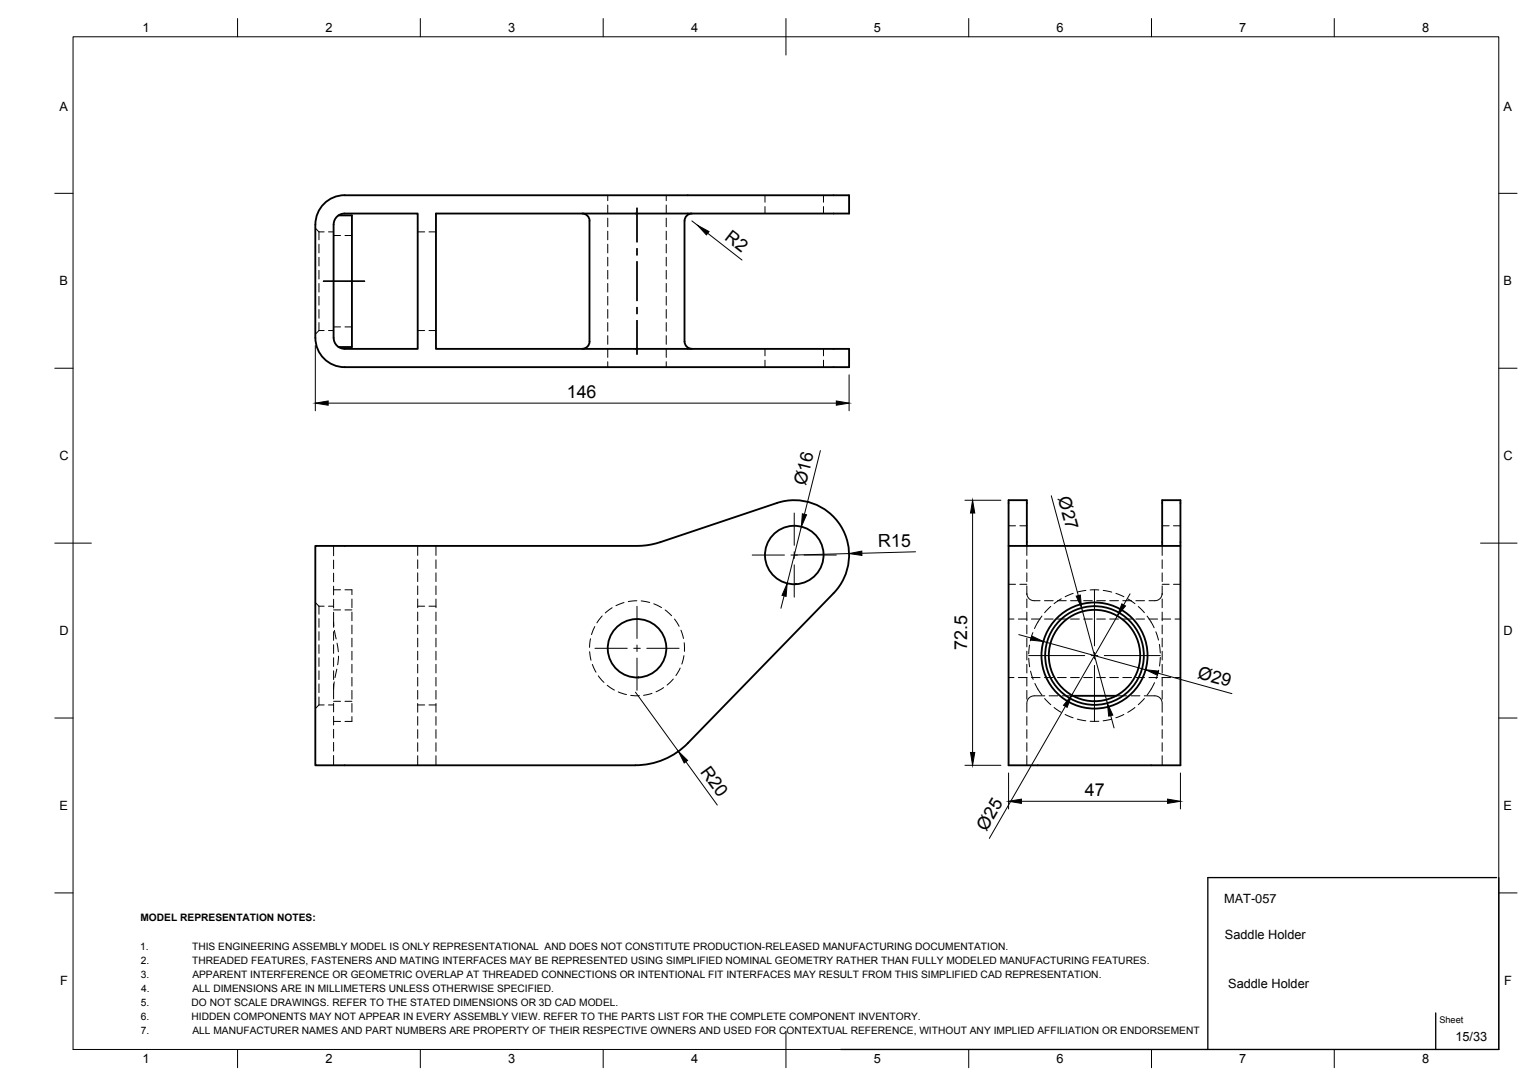
ISO-10303-21;
HEADER;
/* Generated by software containing ST-Developer
 * from STEP Tools, Inc. (www.steptools.com) 
 */

FILE_DESCRIPTION(
/* description */ ('STEP AP214', 'CAx-IF Rec.Pracs.---Representation and Presentation of Product Manufa
cturing Information (PMI)---4.0---2014-10-13'),
/* implementation_level */ '2;1');

FILE_NAME(
/* name */ 'Saddle Holder.step',
/* time_stamp */ '2026-10-28T23:34:22+01:00',
/* author */ (''),
/* organization */ (''),
/* preprocessor_version */ 'ST-DEVELOPER v20.2',
/* originating_system */ 'Autodesk Translation Framework v15.17.0.0',
/* authorisation */ '');

FILE_SCHEMA (('AP242_MANAGED_MODEL_BASED_3D_ENGINEERING_MIM_LF { 1 0 10303 442 2 1 4 }'));
ENDSEC;

DATA;
#10=MECHANICAL_DESIGN_GEOMETRIC_PRESENTATION_REPRESENTATION('',(#255),#27807);
#210=SHAPE_REPRESENTATION_RELATIONSHIP('SRR','None',#27906,#232);
#232=ADVANCED_BREP_SHAPE_REPRESENTATION('',(#284),#27786);
#255=STYLED_ITEM('',(#28091),#284);
#284=MANIFOLD_SOLID_BREP('Body1',#12031);
#378=FACE_BOUND('',#2260,.T.);
#379=FACE_BOUND('',#2261,.T.);
#380=FACE_BOUND('',#2263,.T.);
#381=FACE_BOUND('',#2264,.T.);
#382=FACE_BOUND('',#2266,.T.);
#383=FACE_BOUND('',#2268,.T.);
#384=FACE_BOUND('',#2272,.T.);
#385=FACE_BOUND('',#2276,.T.);
#386=FACE_BOUND('',#2278,.T.);
#387=FACE_BOUND('',#2279,.T.);
#388=FACE_BOUND('',#2281,.T.);
#389=FACE_BOUND('',#2282,.T.);
#390=FACE_BOUND('',#2284,.T.);
#391=FACE_BOUND('',#2289,.T.);
#392=FACE_BOUND('',#2291,.T.);
#559=PLANE('',#12904);
#560=PLANE('',#12908);
#561=PLANE('',#12909);
#562=PLANE('',#12910);
#563=PLANE('',#12913);
#564=PLANE('',#12916);
#565=PLANE('',#12917);
#566=PLANE('',#12920);
#567=PLANE('',#12921);
#568=PLANE('',#12922);
#569=PLANE('',#12927);
#570=PLANE('',#12928);
#571=PLANE('',#12931);
#572=PLANE('',#12934);
#573=PLANE('',#12935);
#574=PLANE('',#12936);
#575=PLANE('',#12937);
#576=PLANE('',#12938);
#577=PLANE('',#12939);
#827=TOROIDAL_SURFACE('',#12863,15.,2.);
#828=TOROIDAL_SURFACE('',#12868,15.,2.);
#874=B_SPLINE_CURVE_WITH_KNOTS('',3,(#19078,#19079,#19080,#19081,#19082,
#19083,#19084,#19085,#19086,#19087,#19088,#19089,#19090,#19091),
 .UNSPECIFIED.,.F.,.F.,(4,2,2,2,2,2,4),(2.17202184366925,2.28922044415962,
2.56626725236737,3.12036086878288,3.67445448519838,3.95150129340613,4.06869989389652),
 .UNSPECIFIED.);
#875=B_SPLINE_CURVE_WITH_KNOTS('',3,(#19095,#19096,#19097,#19098,#19099,
#19100,#19101,#19102),.UNSPECIFIED.,.F.,.F.,(4,2,2,4),(-0.94833902511363,
-0.831140424623256,-0.554093616415504,0.),.UNSPECIFIED.);
#876=B_SPLINE_CURVE_WITH_KNOTS('',3,(#19107,#19108,#19109,#19110,#19111,
#19112,#19113,#19114),.UNSPECIFIED.,.F.,.F.,(4,2,2,4),(0.,0.554093616415503,
0.831140424623253,0.948339025113634),.UNSPECIFIED.);
#1073=CYLINDRICAL_SURFACE('',#12873,13.);
#1074=CYLINDRICAL_SURFACE('',#12874,12.5);
#1075=CYLINDRICAL_SURFACE('',#12877,18.);
#1076=CYLINDRICAL_SURFACE('',#12881,13.5);
#1077=CYLINDRICAL_SURFACE('',#12884,13.5);
#1078=CYLINDRICAL_SURFACE('',#12886,8.00000000000002);
#1079=CYLINDRICAL_SURFACE('',#12889,8.00000000000002);
#1080=CYLINDRICAL_SURFACE('',#12892,15.);
#1081=CYLINDRICAL_SURFACE('',#12895,8.00000000000002);
#1082=CYLINDRICAL_SURFACE('',#12898,15.);
#1083=CYLINDRICAL_SURFACE('',#12901,3.);
#1084=CYLINDRICAL_SURFACE('',#12905,3.);
#1085=CYLINDRICAL_SURFACE('',#12925,8.00000000000001);
#1086=CYLINDRICAL_SURFACE('',#12926,8.00000000000001);
#1087=CYLINDRICAL_SURFACE('',#12940,20.);
#1088=CYLINDRICAL_SURFACE('',#12941,20.);
#1089=CYLINDRICAL_SURFACE('',#12942,20.);
#1090=CYLINDRICAL_SURFACE('',#12943,20.);
#1501=FACE_OUTER_BOUND('',#2241,.T.);
#1502=FACE_OUTER_BOUND('',#2242,.T.);
#1503=FACE_OUTER_BOUND('',#2243,.T.);
#1504=FACE_OUTER_BOUND('',#2244,.T.);
#1505=FACE_OUTER_BOUND('',#2245,.T.);
#1506=FACE_OUTER_BOUND('',#2246,.T.);
#1507=FACE_OUTER_BOUND('',#2247,.T.);
#1508=FACE_OUTER_BOUND('',#2248,.T.);
#1509=FACE_OUTER_BOUND('',#2249,.T.);
#1510=FACE_OUTER_BOUND('',#2250,.T.);
#1511=FACE_OUTER_BOUND('',#2251,.T.);
#1512=FACE_OUTER_BOUND('',#2252,.T.);
#1513=FACE_OUTER_BOUND('',#2253,.T.);
#1514=FACE_OUTER_BOUND('',#2254,.T.);
#1515=FACE_OUTER_BOUND('',#2255,.T.);
#1516=FACE_OUTER_BOUND('',#2256,.T.);
#1517=FACE_OUTER_BOUND('',#2257,.T.);
#1518=FACE_OUTER_BOUND('',#2258,.T.);
#1519=FACE_OUTER_BOUND('',#2259,.T.);
#1520=FACE_OUTER_BOUND('',#2262,.T.);
#1521=FACE_OUTER_BOUND('',#2265,.T.);
#1522=FACE_OUTER_BOUND('',#2267,.T.);
#1523=FACE_OUTER_BOUND('',#2269,.T.);
#1524=FACE_OUTER_BOUND('',#2270,.T.);
#1525=FACE_OUTER_BOUND('',#2271,.T.);
#1526=FACE_OUTER_BOUND('',#2273,.T.);
#1527=FACE_OUTER_BOUND('',#2274,.T.);
#1528=FACE_OUTER_BOUND('',#2275,.T.);
#1529=FACE_OUTER_BOUND('',#2277,.T.);
#1530=FACE_OUTER_BOUND('',#2280,.T.);
#1531=FACE_OUTER_BOUND('',#2283,.T.);
#1532=FACE_OUTER_BOUND('',#2285,.T.);
#1533=FACE_OUTER_BOUND('',#2286,.T.);
#1534=FACE_OUTER_BOUND('',#2287,.T.);
#1535=FACE_OUTER_BOUND('',#2288,.T.);
#1536=FACE_OUTER_BOUND('',#2290,.T.);
#1537=FACE_OUTER_BOUND('',#2292,.T.);
#1538=FACE_OUTER_BOUND('',#2293,.T.);
#1539=FACE_OUTER_BOUND('',#2294,.T.);
#1540=FACE_OUTER_BOUND('',#2295,.T.);
#2241=EDGE_LOOP('',(#9169,#9170,#9171,#9172));
#2242=EDGE_LOOP('',(#9173,#9174,#9175,#9176,#9177));
#2243=EDGE_LOOP('',(#9178,#9179,#9180,#9181,#9182));
#2244=EDGE_LOOP('',(#9183,#9184,#9185,#9186,#9187,#9188));
#2245=EDGE_LOOP('',(#9189,#9190,#9191,#9192));
#2246=EDGE_LOOP('',(#9193,#9194,#9195,#9196,#9197,#9198,#9199,#9200));
#2247=EDGE_LOOP('',(#9201,#9202,#9203,#9204));
#2248=EDGE_LOOP('',(#9205,#9206,#9207,#9208));
#2249=EDGE_LOOP('',(#9209,#9210,#9211,#9212));
#2250=EDGE_LOOP('',(#9213,#9214,#9215,#9216));
#2251=EDGE_LOOP('',(#9217,#9218,#9219,#9220));
#2252=EDGE_LOOP('',(#9221,#9222,#9223,#9224));
#2253=EDGE_LOOP('',(#9225,#9226,#9227,#9228));
#2254=EDGE_LOOP('',(#9229,#9230,#9231,#9232,#9233,#9234));
#2255=EDGE_LOOP('',(#9235,#9236,#9237,#9238));
#2256=EDGE_LOOP('',(#9239,#9240,#9241,#9242,#9243,#9244,#9245));
#2257=EDGE_LOOP('',(#9246,#9247,#9248,#9249));
#2258=EDGE_LOOP('',(#9250,#9251,#9252,#9253));
#2259=EDGE_LOOP('',(#9254,#9255,#9256,#9257,#9258,#9259,#9260,#9261));
#2260=EDGE_LOOP('',(#9262));
#2261=EDGE_LOOP('',(#9263));
#2262=EDGE_LOOP('',(#9264,#9265,#9266,#9267,#9268,#9269,#9270,#9271));
#2263=EDGE_LOOP('',(#9272));
#2264=EDGE_LOOP('',(#9273));
#2265=EDGE_LOOP('',(#9274,#9275,#9276,#9277));
#2266=EDGE_LOOP('',(#9278));
#2267=EDGE_LOOP('',(#9279,#9280,#9281,#9282,#9283,#9284,#9285,#9286,#9287,
#9288));
#2268=EDGE_LOOP('',(#9289,#9290,#9291,#9292,#9293,#9294));
#2269=EDGE_LOOP('',(#9295,#9296,#9297,#9298));
#2270=EDGE_LOOP('',(#9299,#9300,#9301,#9302));
#2271=EDGE_LOOP('',(#9303,#9304,#9305,#9306,#9307,#9308,#9309,#9310,#9311,
#9312));
#2272=EDGE_LOOP('',(#9313,#9314,#9315,#9316,#9317,#9318));
#2273=EDGE_LOOP('',(#9319,#9320,#9321,#9322));
#2274=EDGE_LOOP('',(#9323,#9324,#9325,#9326));
#2275=EDGE_LOOP('',(#9327,#9328,#9329,#9330));
#2276=EDGE_LOOP('',(#9331));
#2277=EDGE_LOOP('',(#9332,#9333,#9334,#9335,#9336,#9337,#9338,#9339));
#2278=EDGE_LOOP('',(#9340));
#2279=EDGE_LOOP('',(#9341));
#2280=EDGE_LOOP('',(#9342,#9343,#9344,#9345,#9346,#9347,#9348,#9349));
#2281=EDGE_LOOP('',(#9350));
#2282=EDGE_LOOP('',(#9351));
#2283=EDGE_LOOP('',(#9352,#9353,#9354,#9355));
#2284=EDGE_LOOP('',(#9356));
#2285=EDGE_LOOP('',(#9357,#9358,#9359,#9360));
#2286=EDGE_LOOP('',(#9361,#9362,#9363,#9364));
#2287=EDGE_LOOP('',(#9365,#9366,#9367,#9368));
#2288=EDGE_LOOP('',(#9369));
#2289=EDGE_LOOP('',(#9370));
#2290=EDGE_LOOP('',(#9371));
#2291=EDGE_LOOP('',(#9372));
#2292=EDGE_LOOP('',(#9373,#9374,#9375,#9376));
#2293=EDGE_LOOP('',(#9377,#9378,#9379,#9380));
#2294=EDGE_LOOP('',(#9381,#9382,#9383,#9384));
#2295=EDGE_LOOP('',(#9385,#9386,#9387,#9388));
#3073=LINE('',#19049,#3893);
#3074=LINE('',#19068,#3894);
#3075=LINE('',#19073,#3895);
#3076=LINE('',#19104,#3896);
#3077=LINE('',#19120,#3897);
#3078=LINE('',#19125,#3898);
#3079=LINE('',#19130,#3899);
#3080=LINE('',#19136,#3900);
#3081=LINE('',#19143,#3901);
#3082=LINE('',#19146,#3902);
#3083=LINE('',#19151,#3903);
#3084=LINE('',#19158,#3904);
#3085=LINE('',#19161,#3905);
#3086=LINE('',#19164,#3906);
#3087=LINE('',#19168,#3907);
#3088=LINE('',#19171,#3908);
#3089=LINE('',#19174,#3909);
#3090=LINE('',#19175,#3910);
#3091=LINE('',#19180,#3911);
#3092=LINE('',#19183,#3912);
#3093=LINE('',#19186,#3913);
#3094=LINE('',#19188,#3914);
#3095=LINE('',#19189,#3915);
#3096=LINE('',#19192,#3916);
#3097=LINE('',#19194,#3917);
#3098=LINE('',#19195,#3918);
#3099=LINE('',#19198,#3919);
#3100=LINE('',#19202,#3920);
#3101=LINE('',#19204,#3921);
#3102=LINE('',#19206,#3922);
#3103=LINE('',#19209,#3923);
#3104=LINE('',#19213,#3924);
#3105=LINE('',#19218,#3925);
#3106=LINE('',#19219,#3926);
#3107=LINE('',#19223,#3927);
#3108=LINE('',#19225,#3928);
#3109=LINE('',#19227,#3929);
#3110=LINE('',#19228,#3930);
#3111=LINE('',#19232,#3931);
#3112=LINE('',#19233,#3932);
#3113=LINE('',#19237,#3933);
#3114=LINE('',#19239,#3934);
#3115=LINE('',#19240,#3935);
#3116=LINE('',#19242,#3936);
#3117=LINE('',#19244,#3937);
#3118=LINE('',#19245,#3938);
#3119=LINE('',#19248,#3939);
#3120=LINE('',#19249,#3940);
#3121=LINE('',#19252,#3941);
#3122=LINE('',#19253,#3942);
#3123=LINE('',#19257,#3943);
#3124=LINE('',#19258,#3944);
#3125=LINE('',#19262,#3945);
#3126=LINE('',#19264,#3946);
#3127=LINE('',#19265,#3947);
#3128=LINE('',#19267,#3948);
#3129=LINE('',#19269,#3949);
#3130=LINE('',#19270,#3950);
#3131=LINE('',#19271,#3951);
#3132=LINE('',#19275,#3952);
#3133=LINE('',#19276,#3953);
#3134=LINE('',#19284,#3954);
#3135=LINE('',#19285,#3955);
#3893=VECTOR('',#15179,13.5);
#3894=VECTOR('',#15204,13.);
#3895=VECTOR('',#15209,12.5);
#3896=VECTOR('',#15216,18.);
#3897=VECTOR('',#15225,13.5);
#3898=VECTOR('',#15232,13.5);
#3899=VECTOR('',#15237,8.00000000000002);
#3900=VECTOR('',#15244,8.00000000000002);
#3901=VECTOR('',#15251,1000.);
#3902=VECTOR('',#15254,1000.);
#3903=VECTOR('',#15259,8.00000000000002);
#3904=VECTOR('',#15266,1000.);
#3905=VECTOR('',#15269,1000.);
#3906=VECTOR('',#15272,1000.);
#3907=VECTOR('',#15275,1000.);
#3908=VECTOR('',#15278,1000.);
#3909=VECTOR('',#15281,1000.);
#3910=VECTOR('',#15282,1000.);
#3911=VECTOR('',#15287,1000.);
#3912=VECTOR('',#15290,1000.);
#3913=VECTOR('',#15293,1000.);
#3914=VECTOR('',#15294,1000.);
#3915=VECTOR('',#15295,1000.);
#3916=VECTOR('',#15298,1000.);
#3917=VECTOR('',#15299,1000.);
#3918=VECTOR('',#15300,1000.);
#3919=VECTOR('',#15303,1000.);
#3920=VECTOR('',#15306,1000.);
#3921=VECTOR('',#15307,1000.);
#3922=VECTOR('',#15308,1000.);
#3923=VECTOR('',#15311,1000.);
#3924=VECTOR('',#15314,1000.);
#3925=VECTOR('',#15319,1000.);
#3926=VECTOR('',#15320,1000.);
#3927=VECTOR('',#15323,1000.);
#3928=VECTOR('',#15324,1000.);
#3929=VECTOR('',#15325,1000.);
#3930=VECTOR('',#15326,1000.);
#3931=VECTOR('',#15329,1000.);
#3932=VECTOR('',#15330,1000.);
#3933=VECTOR('',#15335,1000.);
#3934=VECTOR('',#15336,1000.);
#3935=VECTOR('',#15337,1000.);
#3936=VECTOR('',#15338,1000.);
#3937=VECTOR('',#15339,1000.);
#3938=VECTOR('',#15340,1000.);
#3939=VECTOR('',#15343,1000.);
#3940=VECTOR('',#15344,1000.);
#3941=VECTOR('',#15347,1000.);
#3942=VECTOR('',#15348,1000.);
#3943=VECTOR('',#15351,1000.);
#3944=VECTOR('',#15352,1000.);
#3945=VECTOR('',#15357,1000.);
#3946=VECTOR('',#15358,1000.);
#3947=VECTOR('',#15359,1000.);
#3948=VECTOR('',#15360,1000.);
#3949=VECTOR('',#15361,1000.);
#3950=VECTOR('',#15362,1000.);
#3951=VECTOR('',#15363,1000.);
#3952=VECTOR('',#15370,1000.);
#3953=VECTOR('',#15371,1000.);
#3954=VECTOR('',#15386,1000.);
#3955=VECTOR('',#15387,1000.);
#4669=CIRCLE('',#12861,13.5);
#4670=CIRCLE('',#12862,14.5);
#4671=CIRCLE('',#12864,15.);
#4672=CIRCLE('',#12865,2.);
#4673=CIRCLE('',#12866,13.);
#4674=CIRCLE('',#12867,13.);
#4675=CIRCLE('',#12869,15.);
#4676=CIRCLE('',#12870,2.);
#4677=CIRCLE('',#12871,13.);
#4678=CIRCLE('',#12872,13.);
#4679=CIRCLE('',#12875,12.5);
#4680=CIRCLE('',#12876,12.5);
#4681=CIRCLE('',#12878,18.);
#4682=CIRCLE('',#12879,18.);
#4683=CIRCLE('',#12880,18.);
#4684=CIRCLE('',#12882,13.5);
#4685=CIRCLE('',#12883,13.5);
#4686=CIRCLE('',#12885,13.5);
#4687=CIRCLE('',#12887,8.00000000000002);
#4688=CIRCLE('',#12888,8.00000000000002);
#4689=CIRCLE('',#12890,8.00000000000002);
#4690=CIRCLE('',#12891,8.);
#4691=CIRCLE('',#12893,15.);
#4692=CIRCLE('',#12894,15.);
#4693=CIRCLE('',#12896,7.99999999999999);
#4694=CIRCLE('',#12897,8.00000000000002);
#4695=CIRCLE('',#12899,15.);
#4696=CIRCLE('',#12900,15.);
#4697=CIRCLE('',#12902,3.);
#4698=CIRCLE('',#12903,2.99999999999999);
#4699=CIRCLE('',#12906,2.99999999999999);
#4700=CIRCLE('',#12907,3.);
#4701=CIRCLE('',#12911,20.);
#4702=CIRCLE('',#12912,20.);
#4703=CIRCLE('',#12914,20.);
#4704=CIRCLE('',#12915,20.);
#4705=CIRCLE('',#12918,8.00000000000002);
#4706=CIRCLE('',#12919,8.00000000000002);
#4707=CIRCLE('',#12923,8.00000000000001);
#4708=CIRCLE('',#12924,8.00000000000001);
#4709=CIRCLE('',#12929,20.);
#4710=CIRCLE('',#12930,20.);
#4711=CIRCLE('',#12932,20.);
#4712=CIRCLE('',#12933,20.);
#5461=VERTEX_POINT('',#19046);
#5462=VERTEX_POINT('',#19048);
#5463=VERTEX_POINT('',#19052);
#5464=VERTEX_POINT('',#19054);
#5465=VERTEX_POINT('',#19056);
#5466=VERTEX_POINT('',#19060);
#5467=VERTEX_POINT('',#19062);
#5468=VERTEX_POINT('',#19064);
#5469=VERTEX_POINT('',#19070);
#5470=VERTEX_POINT('',#19072);
#5471=VERTEX_POINT('',#19076);
#5472=VERTEX_POINT('',#19077);
#5473=VERTEX_POINT('',#19092);
#5474=VERTEX_POINT('',#19094);
#5475=VERTEX_POINT('',#19103);
#5476=VERTEX_POINT('',#19106);
#5477=VERTEX_POINT('',#19117);
#5478=VERTEX_POINT('',#19119);
#5479=VERTEX_POINT('',#19123);
#5480=VERTEX_POINT('',#19127);
#5481=VERTEX_POINT('',#19129);
#5482=VERTEX_POINT('',#19133);
#5483=VERTEX_POINT('',#19135);
#5484=VERTEX_POINT('',#19139);
#5485=VERTEX_POINT('',#19140);
#5486=VERTEX_POINT('',#19142);
#5487=VERTEX_POINT('',#19144);
#5488=VERTEX_POINT('',#19148);
#5489=VERTEX_POINT('',#19150);
#5490=VERTEX_POINT('',#19154);
#5491=VERTEX_POINT('',#19155);
#5492=VERTEX_POINT('',#19157);
#5493=VERTEX_POINT('',#19159);
#5494=VERTEX_POINT('',#19163);
#5495=VERTEX_POINT('',#19165);
#5496=VERTEX_POINT('',#19167);
#5497=VERTEX_POINT('',#19169);
#5498=VERTEX_POINT('',#19173);
#5499=VERTEX_POINT('',#19177);
#5500=VERTEX_POINT('',#19179);
#5501=VERTEX_POINT('',#19181);
#5502=VERTEX_POINT('',#19185);
#5503=VERTEX_POINT('',#19187);
#5504=VERTEX_POINT('',#19191);
#5505=VERTEX_POINT('',#19193);
#5506=VERTEX_POINT('',#19197);
#5507=VERTEX_POINT('',#19199);
#5508=VERTEX_POINT('',#19201);
#5509=VERTEX_POINT('',#19203);
#5510=VERTEX_POINT('',#19205);
#5511=VERTEX_POINT('',#19207);
#5512=VERTEX_POINT('',#19211);
#5513=VERTEX_POINT('',#19212);
#5514=VERTEX_POINT('',#19215);
#5515=VERTEX_POINT('',#19217);
#5516=VERTEX_POINT('',#19221);
#5517=VERTEX_POINT('',#19222);
#5518=VERTEX_POINT('',#19224);
#5519=VERTEX_POINT('',#19226);
#5520=VERTEX_POINT('',#19230);
#5521=VERTEX_POINT('',#19231);
#5522=VERTEX_POINT('',#19236);
#5523=VERTEX_POINT('',#19238);
#5524=VERTEX_POINT('',#19241);
#5525=VERTEX_POINT('',#19243);
#5526=VERTEX_POINT('',#19247);
#5527=VERTEX_POINT('',#19251);
#5528=VERTEX_POINT('',#19255);
#5529=VERTEX_POINT('',#19256);
#5530=VERTEX_POINT('',#19261);
#5531=VERTEX_POINT('',#19263);
#5532=VERTEX_POINT('',#19266);
#5533=VERTEX_POINT('',#19268);
#6797=EDGE_CURVE('',#5461,#5461,#4669,.T.);
#6798=EDGE_CURVE('',#5461,#5462,#3073,.T.);
#6799=EDGE_CURVE('',#5462,#5462,#4670,.T.);
#6800=EDGE_CURVE('',#5463,#5463,#4671,.T.);
#6801=EDGE_CURVE('',#5463,#5464,#4672,.T.);
#6802=EDGE_CURVE('',#5465,#5464,#4673,.T.);
#6803=EDGE_CURVE('',#5464,#5465,#4674,.T.);
#6804=EDGE_CURVE('',#5466,#5466,#4675,.T.);
#6805=EDGE_CURVE('',#5466,#5467,#4676,.T.);
#6806=EDGE_CURVE('',#5468,#5467,#4677,.T.);
#6807=EDGE_CURVE('',#5467,#5468,#4678,.T.);
#6808=EDGE_CURVE('',#5465,#5468,#3074,.T.);
#6809=EDGE_CURVE('',#5469,#5469,#4679,.T.);
#6810=EDGE_CURVE('',#5469,#5470,#3075,.T.);
#6811=EDGE_CURVE('',#5470,#5470,#4680,.T.);
#6812=EDGE_CURVE('',#5471,#5472,#874,.F.);
#6813=EDGE_CURVE('',#5472,#5473,#4681,.T.);
#6814=EDGE_CURVE('',#5473,#5474,#875,.T.);
#6815=EDGE_CURVE('',#5474,#5475,#3076,.T.);
#6816=EDGE_CURVE('',#5475,#5475,#4682,.T.);
#6817=EDGE_CURVE('',#5474,#5476,#876,.T.);
#6818=EDGE_CURVE('',#5476,#5471,#4683,.T.);
#6819=EDGE_CURVE('',#5477,#5477,#4684,.T.);
#6820=EDGE_CURVE('',#5477,#5478,#3077,.T.);
#6821=EDGE_CURVE('',#5478,#5478,#4685,.T.);
#6822=EDGE_CURVE('',#5479,#5479,#4686,.T.);
#6823=EDGE_CURVE('',#5479,#5461,#3078,.T.);
#6824=EDGE_CURVE('',#5480,#5480,#4687,.T.);
#6825=EDGE_CURVE('',#5480,#5481,#3079,.T.);
#6826=EDGE_CURVE('',#5481,#5481,#4688,.T.);
#6827=EDGE_CURVE('',#5482,#5482,#4689,.T.);
#6828=EDGE_CURVE('',#5482,#5483,#3080,.T.);
#6829=EDGE_CURVE('',#5483,#5483,#4690,.T.);
#6830=EDGE_CURVE('',#5484,#5485,#4691,.T.);
#6831=EDGE_CURVE('',#5485,#5486,#3081,.T.);
#6832=EDGE_CURVE('',#5486,#5487,#4692,.T.);
#6833=EDGE_CURVE('',#5484,#5487,#3082,.T.);
#6834=EDGE_CURVE('',#5488,#5488,#4693,.T.);
#6835=EDGE_CURVE('',#5488,#5489,#3083,.T.);
#6836=EDGE_CURVE('',#5489,#5489,#4694,.T.);
#6837=EDGE_CURVE('',#5490,#5491,#4695,.T.);
#6838=EDGE_CURVE('',#5490,#5492,#3084,.T.);
#6839=EDGE_CURVE('',#5492,#5493,#4696,.T.);
#6840=EDGE_CURVE('',#5491,#5493,#3085,.T.);
#6841=EDGE_CURVE('',#5471,#5494,#3086,.T.);
#6842=EDGE_CURVE('',#5494,#5495,#4697,.T.);
#6843=EDGE_CURVE('',#5496,#5495,#3087,.T.);
#6844=EDGE_CURVE('',#5497,#5496,#4698,.T.);
#6845=EDGE_CURVE('',#5497,#5472,#3088,.T.);
#6846=EDGE_CURVE('',#5498,#5497,#3089,.T.);
#6847=EDGE_CURVE('',#5498,#5473,#3090,.T.);
#6848=EDGE_CURVE('',#5499,#5498,#4699,.T.);
#6849=EDGE_CURVE('',#5499,#5500,#3091,.T.);
#6850=EDGE_CURVE('',#5500,#5501,#4700,.T.);
#6851=EDGE_CURVE('',#5476,#5501,#3092,.T.);
#6852=EDGE_CURVE('',#5485,#5502,#3093,.T.);
#6853=EDGE_CURVE('',#5502,#5503,#3094,.T.);
#6854=EDGE_CURVE('',#5503,#5486,#3095,.T.);
#6855=EDGE_CURVE('',#5487,#5504,#3096,.T.);
#6856=EDGE_CURVE('',#5504,#5505,#3097,.T.);
#6857=EDGE_CURVE('',#5505,#5484,#3098,.T.);
#6858=EDGE_CURVE('',#5491,#5506,#3099,.T.);
#6859=EDGE_CURVE('',#5506,#5507,#4701,.T.);
#6860=EDGE_CURVE('',#5507,#5508,#3100,.T.);
#6861=EDGE_CURVE('',#5508,#5509,#3101,.T.);
#6862=EDGE_CURVE('',#5509,#5510,#3102,.T.);
#6863=EDGE_CURVE('',#5510,#5511,#4702,.T.);
#6864=EDGE_CURVE('',#5511,#5490,#3103,.T.);
#6865=EDGE_CURVE('',#5512,#5513,#3104,.T.);
#6866=EDGE_CURVE('',#5512,#5504,#4703,.T.);
#6867=EDGE_CURVE('',#5503,#5514,#4704,.T.);
#6868=EDGE_CURVE('',#5515,#5514,#3105,.T.);
#6869=EDGE_CURVE('',#5515,#5513,#3106,.T.);
#6870=EDGE_CURVE('',#5516,#5517,#3107,.T.);
#6871=EDGE_CURVE('',#5517,#5518,#3108,.T.);
#6872=EDGE_CURVE('',#5519,#5518,#3109,.T.);
#6873=EDGE_CURVE('',#5519,#5516,#3110,.T.);
#6874=EDGE_CURVE('',#5520,#5521,#3111,.T.);
#6875=EDGE_CURVE('',#5521,#5510,#3112,.T.);
#6876=EDGE_CURVE('',#5509,#5519,#4705,.T.);
#6877=EDGE_CURVE('',#5518,#5515,#4706,.T.);
#6878=EDGE_CURVE('',#5514,#5522,#3113,.T.);
#6879=EDGE_CURVE('',#5522,#5523,#3114,.T.);
#6880=EDGE_CURVE('',#5523,#5520,#3115,.T.);
#6881=EDGE_CURVE('',#5496,#5524,#3116,.T.);
#6882=EDGE_CURVE('',#5524,#5525,#3117,.T.);
#6883=EDGE_CURVE('',#5525,#5499,#3118,.T.);
#6884=EDGE_CURVE('',#5511,#5526,#3119,.T.);
#6885=EDGE_CURVE('',#5526,#5492,#3120,.T.);
#6886=EDGE_CURVE('',#5493,#5527,#3121,.T.);
#6887=EDGE_CURVE('',#5527,#5506,#3122,.T.);
#6888=EDGE_CURVE('',#5528,#5529,#3123,.T.);
#6889=EDGE_CURVE('',#5528,#5512,#3124,.T.);
#6890=EDGE_CURVE('',#5513,#5517,#4707,.T.);
#6891=EDGE_CURVE('',#5516,#5508,#4708,.T.);
#6892=EDGE_CURVE('',#5507,#5530,#3125,.T.);
#6893=EDGE_CURVE('',#5531,#5530,#3126,.T.);
#6894=EDGE_CURVE('',#5529,#5531,#3127,.T.);
#6895=EDGE_CURVE('',#5532,#5500,#3128,.T.);
#6896=EDGE_CURVE('',#5533,#5532,#3129,.T.);
#6897=EDGE_CURVE('',#5495,#5533,#3130,.T.);
#6898=EDGE_CURVE('',#5501,#5494,#3131,.T.);
#6899=EDGE_CURVE('',#5523,#5529,#3132,.T.);
#6900=EDGE_CURVE('',#5520,#5531,#3133,.T.);
#6901=EDGE_CURVE('',#5505,#5528,#4709,.T.);
#6902=EDGE_CURVE('',#5522,#5502,#4710,.T.);
#6903=EDGE_CURVE('',#5530,#5527,#4711,.T.);
#6904=EDGE_CURVE('',#5526,#5521,#4712,.T.);
#6905=EDGE_CURVE('',#5524,#5533,#3134,.T.);
#6906=EDGE_CURVE('',#5525,#5532,#3135,.T.);
#9169=ORIENTED_EDGE('',*,*,#6797,.F.);
#9170=ORIENTED_EDGE('',*,*,#6798,.T.);
#9171=ORIENTED_EDGE('',*,*,#6799,.F.);
#9172=ORIENTED_EDGE('',*,*,#6798,.F.);
#9173=ORIENTED_EDGE('',*,*,#6800,.F.);
#9174=ORIENTED_EDGE('',*,*,#6801,.T.);
#9175=ORIENTED_EDGE('',*,*,#6802,.F.);
#9176=ORIENTED_EDGE('',*,*,#6803,.F.);
#9177=ORIENTED_EDGE('',*,*,#6801,.F.);
#9178=ORIENTED_EDGE('',*,*,#6804,.F.);
#9179=ORIENTED_EDGE('',*,*,#6805,.T.);
#9180=ORIENTED_EDGE('',*,*,#6806,.F.);
#9181=ORIENTED_EDGE('',*,*,#6807,.F.);
#9182=ORIENTED_EDGE('',*,*,#6805,.F.);
#9183=ORIENTED_EDGE('',*,*,#6802,.T.);
#9184=ORIENTED_EDGE('',*,*,#6803,.T.);
#9185=ORIENTED_EDGE('',*,*,#6808,.T.);
#9186=ORIENTED_EDGE('',*,*,#6806,.T.);
#9187=ORIENTED_EDGE('',*,*,#6807,.T.);
#9188=ORIENTED_EDGE('',*,*,#6808,.F.);
#9189=ORIENTED_EDGE('',*,*,#6809,.T.);
#9190=ORIENTED_EDGE('',*,*,#6810,.T.);
#9191=ORIENTED_EDGE('',*,*,#6811,.F.);
#9192=ORIENTED_EDGE('',*,*,#6810,.F.);
#9193=ORIENTED_EDGE('',*,*,#6812,.T.);
#9194=ORIENTED_EDGE('',*,*,#6813,.T.);
#9195=ORIENTED_EDGE('',*,*,#6814,.T.);
#9196=ORIENTED_EDGE('',*,*,#6815,.T.);
#9197=ORIENTED_EDGE('',*,*,#6816,.F.);
#9198=ORIENTED_EDGE('',*,*,#6815,.F.);
#9199=ORIENTED_EDGE('',*,*,#6817,.T.);
#9200=ORIENTED_EDGE('',*,*,#6818,.T.);
#9201=ORIENTED_EDGE('',*,*,#6819,.T.);
#9202=ORIENTED_EDGE('',*,*,#6820,.T.);
#9203=ORIENTED_EDGE('',*,*,#6821,.F.);
#9204=ORIENTED_EDGE('',*,*,#6820,.F.);
#9205=ORIENTED_EDGE('',*,*,#6822,.F.);
#9206=ORIENTED_EDGE('',*,*,#6823,.T.);
#9207=ORIENTED_EDGE('',*,*,#6797,.T.);
#9208=ORIENTED_EDGE('',*,*,#6823,.F.);
#9209=ORIENTED_EDGE('',*,*,#6824,.T.);
#9210=ORIENTED_EDGE('',*,*,#6825,.T.);
#9211=ORIENTED_EDGE('',*,*,#6826,.F.);
#9212=ORIENTED_EDGE('',*,*,#6825,.F.);
#9213=ORIENTED_EDGE('',*,*,#6827,.T.);
#9214=ORIENTED_EDGE('',*,*,#6828,.T.);
#9215=ORIENTED_EDGE('',*,*,#6829,.F.);
#9216=ORIENTED_EDGE('',*,*,#6828,.F.);
#9217=ORIENTED_EDGE('',*,*,#6830,.T.);
#9218=ORIENTED_EDGE('',*,*,#6831,.T.);
#9219=ORIENTED_EDGE('',*,*,#6832,.T.);
#9220=ORIENTED_EDGE('',*,*,#6833,.F.);
#9221=ORIENTED_EDGE('',*,*,#6834,.F.);
#9222=ORIENTED_EDGE('',*,*,#6835,.T.);
#9223=ORIENTED_EDGE('',*,*,#6836,.F.);
#9224=ORIENTED_EDGE('',*,*,#6835,.F.);
#9225=ORIENTED_EDGE('',*,*,#6837,.F.);
#9226=ORIENTED_EDGE('',*,*,#6838,.T.);
#9227=ORIENTED_EDGE('',*,*,#6839,.T.);
#9228=ORIENTED_EDGE('',*,*,#6840,.F.);
#9229=ORIENTED_EDGE('',*,*,#6812,.F.);
#9230=ORIENTED_EDGE('',*,*,#6841,.T.);
#9231=ORIENTED_EDGE('',*,*,#6842,.T.);
#9232=ORIENTED_EDGE('',*,*,#6843,.F.);
#9233=ORIENTED_EDGE('',*,*,#6844,.F.);
#9234=ORIENTED_EDGE('',*,*,#6845,.T.);
#9235=ORIENTED_EDGE('',*,*,#6813,.F.);
#9236=ORIENTED_EDGE('',*,*,#6845,.F.);
#9237=ORIENTED_EDGE('',*,*,#6846,.F.);
#9238=ORIENTED_EDGE('',*,*,#6847,.T.);
#9239=ORIENTED_EDGE('',*,*,#6814,.F.);
#9240=ORIENTED_EDGE('',*,*,#6847,.F.);
#9241=ORIENTED_EDGE('',*,*,#6848,.F.);
#9242=ORIENTED_EDGE('',*,*,#6849,.T.);
#9243=ORIENTED_EDGE('',*,*,#6850,.T.);
#9244=ORIENTED_EDGE('',*,*,#6851,.F.);
#9245=ORIENTED_EDGE('',*,*,#6817,.F.);
#9246=ORIENTED_EDGE('',*,*,#6852,.T.);
#9247=ORIENTED_EDGE('',*,*,#6853,.T.);
#9248=ORIENTED_EDGE('',*,*,#6854,.T.);
#9249=ORIENTED_EDGE('',*,*,#6831,.F.);
#9250=ORIENTED_EDGE('',*,*,#6855,.T.);
#9251=ORIENTED_EDGE('',*,*,#6856,.T.);
#9252=ORIENTED_EDGE('',*,*,#6857,.T.);
#9253=ORIENTED_EDGE('',*,*,#6833,.T.);
#9254=ORIENTED_EDGE('',*,*,#6858,.T.);
#9255=ORIENTED_EDGE('',*,*,#6859,.T.);
#9256=ORIENTED_EDGE('',*,*,#6860,.T.);
#9257=ORIENTED_EDGE('',*,*,#6861,.T.);
#9258=ORIENTED_EDGE('',*,*,#6862,.T.);
#9259=ORIENTED_EDGE('',*,*,#6863,.T.);
#9260=ORIENTED_EDGE('',*,*,#6864,.T.);
#9261=ORIENTED_EDGE('',*,*,#6837,.T.);
#9262=ORIENTED_EDGE('',*,*,#6824,.F.);
#9263=ORIENTED_EDGE('',*,*,#6827,.F.);
#9264=ORIENTED_EDGE('',*,*,#6865,.F.);
#9265=ORIENTED_EDGE('',*,*,#6866,.T.);
#9266=ORIENTED_EDGE('',*,*,#6855,.F.);
#9267=ORIENTED_EDGE('',*,*,#6832,.F.);
#9268=ORIENTED_EDGE('',*,*,#6854,.F.);
#9269=ORIENTED_EDGE('',*,*,#6867,.T.);
#9270=ORIENTED_EDGE('',*,*,#6868,.F.);
#9271=ORIENTED_EDGE('',*,*,#6869,.T.);
#9272=ORIENTED_EDGE('',*,*,#6836,.T.);
#9273=ORIENTED_EDGE('',*,*,#6826,.T.);
#9274=ORIENTED_EDGE('',*,*,#6870,.T.);
#9275=ORIENTED_EDGE('',*,*,#6871,.T.);
#9276=ORIENTED_EDGE('',*,*,#6872,.F.);
#9277=ORIENTED_EDGE('',*,*,#6873,.T.);
#9278=ORIENTED_EDGE('',*,*,#6799,.T.);
#9279=ORIENTED_EDGE('',*,*,#6874,.T.);
#9280=ORIENTED_EDGE('',*,*,#6875,.T.);
#9281=ORIENTED_EDGE('',*,*,#6862,.F.);
#9282=ORIENTED_EDGE('',*,*,#6876,.T.);
#9283=ORIENTED_EDGE('',*,*,#6872,.T.);
#9284=ORIENTED_EDGE('',*,*,#6877,.T.);
#9285=ORIENTED_EDGE('',*,*,#6868,.T.);
#9286=ORIENTED_EDGE('',*,*,#6878,.T.);
#9287=ORIENTED_EDGE('',*,*,#6879,.T.);
#9288=ORIENTED_EDGE('',*,*,#6880,.T.);
#9289=ORIENTED_EDGE('',*,*,#6881,.T.);
#9290=ORIENTED_EDGE('',*,*,#6882,.T.);
#9291=ORIENTED_EDGE('',*,*,#6883,.T.);
#9292=ORIENTED_EDGE('',*,*,#6848,.T.);
#9293=ORIENTED_EDGE('',*,*,#6846,.T.);
#9294=ORIENTED_EDGE('',*,*,#6844,.T.);
#9295=ORIENTED_EDGE('',*,*,#6864,.F.);
#9296=ORIENTED_EDGE('',*,*,#6884,.T.);
#9297=ORIENTED_EDGE('',*,*,#6885,.T.);
#9298=ORIENTED_EDGE('',*,*,#6838,.F.);
#9299=ORIENTED_EDGE('',*,*,#6886,.T.);
#9300=ORIENTED_EDGE('',*,*,#6887,.T.);
#9301=ORIENTED_EDGE('',*,*,#6858,.F.);
#9302=ORIENTED_EDGE('',*,*,#6840,.T.);
#9303=ORIENTED_EDGE('',*,*,#6888,.F.);
#9304=ORIENTED_EDGE('',*,*,#6889,.T.);
#9305=ORIENTED_EDGE('',*,*,#6865,.T.);
#9306=ORIENTED_EDGE('',*,*,#6890,.T.);
#9307=ORIENTED_EDGE('',*,*,#6870,.F.);
#9308=ORIENTED_EDGE('',*,*,#6891,.T.);
#9309=ORIENTED_EDGE('',*,*,#6860,.F.);
#9310=ORIENTED_EDGE('',*,*,#6892,.T.);
#9311=ORIENTED_EDGE('',*,*,#6893,.F.);
#9312=ORIENTED_EDGE('',*,*,#6894,.F.);
#9313=ORIENTED_EDGE('',*,*,#6895,.F.);
#9314=ORIENTED_EDGE('',*,*,#6896,.F.);
#9315=ORIENTED_EDGE('',*,*,#6897,.F.);
#9316=ORIENTED_EDGE('',*,*,#6842,.F.);
#9317=ORIENTED_EDGE('',*,*,#6898,.F.);
#9318=ORIENTED_EDGE('',*,*,#6850,.F.);
#9319=ORIENTED_EDGE('',*,*,#6890,.F.);
#9320=ORIENTED_EDGE('',*,*,#6869,.F.);
#9321=ORIENTED_EDGE('',*,*,#6877,.F.);
#9322=ORIENTED_EDGE('',*,*,#6871,.F.);
#9323=ORIENTED_EDGE('',*,*,#6891,.F.);
#9324=ORIENTED_EDGE('',*,*,#6873,.F.);
#9325=ORIENTED_EDGE('',*,*,#6876,.F.);
#9326=ORIENTED_EDGE('',*,*,#6861,.F.);
#9327=ORIENTED_EDGE('',*,*,#6899,.T.);
#9328=ORIENTED_EDGE('',*,*,#6894,.T.);
#9329=ORIENTED_EDGE('',*,*,#6900,.F.);
#9330=ORIENTED_EDGE('',*,*,#6880,.F.);
#9331=ORIENTED_EDGE('',*,*,#6819,.F.);
#9332=ORIENTED_EDGE('',*,*,#6857,.F.);
#9333=ORIENTED_EDGE('',*,*,#6901,.T.);
#9334=ORIENTED_EDGE('',*,*,#6888,.T.);
#9335=ORIENTED_EDGE('',*,*,#6899,.F.);
#9336=ORIENTED_EDGE('',*,*,#6879,.F.);
#9337=ORIENTED_EDGE('',*,*,#6902,.T.);
#9338=ORIENTED_EDGE('',*,*,#6852,.F.);
#9339=ORIENTED_EDGE('',*,*,#6830,.F.);
#9340=ORIENTED_EDGE('',*,*,#6800,.T.);
#9341=ORIENTED_EDGE('',*,*,#6834,.T.);
#9342=ORIENTED_EDGE('',*,*,#6893,.T.);
#9343=ORIENTED_EDGE('',*,*,#6903,.T.);
#9344=ORIENTED_EDGE('',*,*,#6886,.F.);
#9345=ORIENTED_EDGE('',*,*,#6839,.F.);
#9346=ORIENTED_EDGE('',*,*,#6885,.F.);
#9347=ORIENTED_EDGE('',*,*,#6904,.T.);
#9348=ORIENTED_EDGE('',*,*,#6874,.F.);
#9349=ORIENTED_EDGE('',*,*,#6900,.T.);
#9350=ORIENTED_EDGE('',*,*,#6804,.T.);
#9351=ORIENTED_EDGE('',*,*,#6829,.T.);
#9352=ORIENTED_EDGE('',*,*,#6905,.T.);
#9353=ORIENTED_EDGE('',*,*,#6896,.T.);
#9354=ORIENTED_EDGE('',*,*,#6906,.F.);
#9355=ORIENTED_EDGE('',*,*,#6882,.F.);
#9356=ORIENTED_EDGE('',*,*,#6821,.T.);
#9357=ORIENTED_EDGE('',*,*,#6843,.T.);
#9358=ORIENTED_EDGE('',*,*,#6897,.T.);
#9359=ORIENTED_EDGE('',*,*,#6905,.F.);
#9360=ORIENTED_EDGE('',*,*,#6881,.F.);
#9361=ORIENTED_EDGE('',*,*,#6818,.F.);
#9362=ORIENTED_EDGE('',*,*,#6851,.T.);
#9363=ORIENTED_EDGE('',*,*,#6898,.T.);
#9364=ORIENTED_EDGE('',*,*,#6841,.F.);
#9365=ORIENTED_EDGE('',*,*,#6906,.T.);
#9366=ORIENTED_EDGE('',*,*,#6895,.T.);
#9367=ORIENTED_EDGE('',*,*,#6849,.F.);
#9368=ORIENTED_EDGE('',*,*,#6883,.F.);
#9369=ORIENTED_EDGE('',*,*,#6822,.T.);
#9370=ORIENTED_EDGE('',*,*,#6811,.T.);
#9371=ORIENTED_EDGE('',*,*,#6816,.T.);
#9372=ORIENTED_EDGE('',*,*,#6809,.F.);
#9373=ORIENTED_EDGE('',*,*,#6863,.F.);
#9374=ORIENTED_EDGE('',*,*,#6875,.F.);
#9375=ORIENTED_EDGE('',*,*,#6904,.F.);
#9376=ORIENTED_EDGE('',*,*,#6884,.F.);
#9377=ORIENTED_EDGE('',*,*,#6902,.F.);
#9378=ORIENTED_EDGE('',*,*,#6878,.F.);
#9379=ORIENTED_EDGE('',*,*,#6867,.F.);
#9380=ORIENTED_EDGE('',*,*,#6853,.F.);
#9381=ORIENTED_EDGE('',*,*,#6901,.F.);
#9382=ORIENTED_EDGE('',*,*,#6856,.F.);
#9383=ORIENTED_EDGE('',*,*,#6866,.F.);
#9384=ORIENTED_EDGE('',*,*,#6889,.F.);
#9385=ORIENTED_EDGE('',*,*,#6859,.F.);
#9386=ORIENTED_EDGE('',*,*,#6887,.F.);
#9387=ORIENTED_EDGE('',*,*,#6903,.F.);
#9388=ORIENTED_EDGE('',*,*,#6892,.F.);
#11300=CONICAL_SURFACE('',#12860,13.5,0.785398163397453);
#11583=ADVANCED_FACE('',(#1501),#11300,.F.);
#11584=ADVANCED_FACE('',(#1502),#827,.F.);
#11585=ADVANCED_FACE('',(#1503),#828,.F.);
#11586=ADVANCED_FACE('',(#1504),#1073,.T.);
#11587=ADVANCED_FACE('',(#1505),#1074,.F.);
#11588=ADVANCED_FACE('',(#1506),#1075,.T.);
#11589=ADVANCED_FACE('',(#1507),#1076,.F.);
#11590=ADVANCED_FACE('',(#1508),#1077,.F.);
#11591=ADVANCED_FACE('',(#1509),#1078,.F.);
#11592=ADVANCED_FACE('',(#1510),#1079,.F.);
#11593=ADVANCED_FACE('',(#1511),#1080,.T.);
#11594=ADVANCED_FACE('',(#1512),#1081,.F.);
#11595=ADVANCED_FACE('',(#1513),#1082,.T.);
#11596=ADVANCED_FACE('',(#1514),#1083,.F.);
#11597=ADVANCED_FACE('',(#1515),#559,.F.);
#11598=ADVANCED_FACE('',(#1516),#1084,.F.);
#11599=ADVANCED_FACE('',(#1517),#560,.F.);
#11600=ADVANCED_FACE('',(#1518),#561,.F.);
#11601=ADVANCED_FACE('',(#1519,#378,#379),#562,.T.);
#11602=ADVANCED_FACE('',(#1520,#380,#381),#563,.F.);
#11603=ADVANCED_FACE('',(#1521,#382),#564,.F.);
#11604=ADVANCED_FACE('',(#1522,#383),#565,.F.);
#11605=ADVANCED_FACE('',(#1523),#566,.F.);
#11606=ADVANCED_FACE('',(#1524),#567,.F.);
#11607=ADVANCED_FACE('',(#1525,#384),#568,.F.);
#11608=ADVANCED_FACE('',(#1526),#1085,.T.);
#11609=ADVANCED_FACE('',(#1527),#1086,.T.);
#11610=ADVANCED_FACE('',(#1528,#385),#569,.F.);
#11611=ADVANCED_FACE('',(#1529,#386,#387),#570,.F.);
#11612=ADVANCED_FACE('',(#1530,#388,#389),#571,.F.);
#11613=ADVANCED_FACE('',(#1531,#390),#572,.F.);
#11614=ADVANCED_FACE('',(#1532),#573,.F.);
#11615=ADVANCED_FACE('',(#1533),#574,.F.);
#11616=ADVANCED_FACE('',(#1534),#575,.F.);
#11617=ADVANCED_FACE('',(#1535,#391),#576,.F.);
#11618=ADVANCED_FACE('',(#1536,#392),#577,.T.);
#11619=ADVANCED_FACE('',(#1537),#1087,.F.);
#11620=ADVANCED_FACE('',(#1538),#1088,.F.);
#11621=ADVANCED_FACE('',(#1539),#1089,.T.);
#11622=ADVANCED_FACE('',(#1540),#1090,.T.);
#12031=CLOSED_SHELL('',(#11583,#11584,#11585,#11586,#11587,#11588,#11589,
#11590,#11591,#11592,#11593,#11594,#11595,#11596,#11597,#11598,#11599,#11600,
#11601,#11602,#11603,#11604,#11605,#11606,#11607,#11608,#11609,#11610,#11611,
#11612,#11613,#11614,#11615,#11616,#11617,#11618,#11619,#11620,#11621,#11622));
#12859=AXIS2_PLACEMENT_3D('',#19044,#15173,#15174);
#12860=AXIS2_PLACEMENT_3D('',#19045,#15175,#15176);
#12861=AXIS2_PLACEMENT_3D('',#19047,#15177,#15178);
#12862=AXIS2_PLACEMENT_3D('',#19050,#15180,#15181);
#12863=AXIS2_PLACEMENT_3D('',#19051,#15182,#15183);
#12864=AXIS2_PLACEMENT_3D('',#19053,#15184,#15185);
#12865=AXIS2_PLACEMENT_3D('',#19055,#15186,#15187);
#12866=AXIS2_PLACEMENT_3D('',#19057,#15188,#15189);
#12867=AXIS2_PLACEMENT_3D('',#19058,#15190,#15191);
#12868=AXIS2_PLACEMENT_3D('',#19059,#15192,#15193);
#12869=AXIS2_PLACEMENT_3D('',#19061,#15194,#15195);
#12870=AXIS2_PLACEMENT_3D('',#19063,#15196,#15197);
#12871=AXIS2_PLACEMENT_3D('',#19065,#15198,#15199);
#12872=AXIS2_PLACEMENT_3D('',#19066,#15200,#15201);
#12873=AXIS2_PLACEMENT_3D('',#19067,#15202,#15203);
#12874=AXIS2_PLACEMENT_3D('',#19069,#15205,#15206);
#12875=AXIS2_PLACEMENT_3D('',#19071,#15207,#15208);
#12876=AXIS2_PLACEMENT_3D('',#19074,#15210,#15211);
#12877=AXIS2_PLACEMENT_3D('',#19075,#15212,#15213);
#12878=AXIS2_PLACEMENT_3D('',#19093,#15214,#15215);
#12879=AXIS2_PLACEMENT_3D('',#19105,#15217,#15218);
#12880=AXIS2_PLACEMENT_3D('',#19115,#15219,#15220);
#12881=AXIS2_PLACEMENT_3D('',#19116,#15221,#15222);
#12882=AXIS2_PLACEMENT_3D('',#19118,#15223,#15224);
#12883=AXIS2_PLACEMENT_3D('',#19121,#15226,#15227);
#12884=AXIS2_PLACEMENT_3D('',#19122,#15228,#15229);
#12885=AXIS2_PLACEMENT_3D('',#19124,#15230,#15231);
#12886=AXIS2_PLACEMENT_3D('',#19126,#15233,#15234);
#12887=AXIS2_PLACEMENT_3D('',#19128,#15235,#15236);
#12888=AXIS2_PLACEMENT_3D('',#19131,#15238,#15239);
#12889=AXIS2_PLACEMENT_3D('',#19132,#15240,#15241);
#12890=AXIS2_PLACEMENT_3D('',#19134,#15242,#15243);
#12891=AXIS2_PLACEMENT_3D('',#19137,#15245,#15246);
#12892=AXIS2_PLACEMENT_3D('',#19138,#15247,#15248);
#12893=AXIS2_PLACEMENT_3D('',#19141,#15249,#15250);
#12894=AXIS2_PLACEMENT_3D('',#19145,#15252,#15253);
#12895=AXIS2_PLACEMENT_3D('',#19147,#15255,#15256);
#12896=AXIS2_PLACEMENT_3D('',#19149,#15257,#15258);
#12897=AXIS2_PLACEMENT_3D('',#19152,#15260,#15261);
#12898=AXIS2_PLACEMENT_3D('',#19153,#15262,#15263);
#12899=AXIS2_PLACEMENT_3D('',#19156,#15264,#15265);
#12900=AXIS2_PLACEMENT_3D('',#19160,#15267,#15268);
#12901=AXIS2_PLACEMENT_3D('',#19162,#15270,#15271);
#12902=AXIS2_PLACEMENT_3D('',#19166,#15273,#15274);
#12903=AXIS2_PLACEMENT_3D('',#19170,#15276,#15277);
#12904=AXIS2_PLACEMENT_3D('',#19172,#15279,#15280);
#12905=AXIS2_PLACEMENT_3D('',#19176,#15283,#15284);
#12906=AXIS2_PLACEMENT_3D('',#19178,#15285,#15286);
#12907=AXIS2_PLACEMENT_3D('',#19182,#15288,#15289);
#12908=AXIS2_PLACEMENT_3D('',#19184,#15291,#15292);
#12909=AXIS2_PLACEMENT_3D('',#19190,#15296,#15297);
#12910=AXIS2_PLACEMENT_3D('',#19196,#15301,#15302);
#12911=AXIS2_PLACEMENT_3D('',#19200,#15304,#15305);
#12912=AXIS2_PLACEMENT_3D('',#19208,#15309,#15310);
#12913=AXIS2_PLACEMENT_3D('',#19210,#15312,#15313);
#12914=AXIS2_PLACEMENT_3D('',#19214,#15315,#15316);
#12915=AXIS2_PLACEMENT_3D('',#19216,#15317,#15318);
#12916=AXIS2_PLACEMENT_3D('',#19220,#15321,#15322);
#12917=AXIS2_PLACEMENT_3D('',#19229,#15327,#15328);
#12918=AXIS2_PLACEMENT_3D('',#19234,#15331,#15332);
#12919=AXIS2_PLACEMENT_3D('',#19235,#15333,#15334);
#12920=AXIS2_PLACEMENT_3D('',#19246,#15341,#15342);
#12921=AXIS2_PLACEMENT_3D('',#19250,#15345,#15346);
#12922=AXIS2_PLACEMENT_3D('',#19254,#15349,#15350);
#12923=AXIS2_PLACEMENT_3D('',#19259,#15353,#15354);
#12924=AXIS2_PLACEMENT_3D('',#19260,#15355,#15356);
#12925=AXIS2_PLACEMENT_3D('',#19272,#15364,#15365);
#12926=AXIS2_PLACEMENT_3D('',#19273,#15366,#15367);
#12927=AXIS2_PLACEMENT_3D('',#19274,#15368,#15369);
#12928=AXIS2_PLACEMENT_3D('',#19277,#15372,#15373);
#12929=AXIS2_PLACEMENT_3D('',#19278,#15374,#15375);
#12930=AXIS2_PLACEMENT_3D('',#19279,#15376,#15377);
#12931=AXIS2_PLACEMENT_3D('',#19280,#15378,#15379);
#12932=AXIS2_PLACEMENT_3D('',#19281,#15380,#15381);
#12933=AXIS2_PLACEMENT_3D('',#19282,#15382,#15383);
#12934=AXIS2_PLACEMENT_3D('',#19283,#15384,#15385);
#12935=AXIS2_PLACEMENT_3D('',#19286,#15388,#15389);
#12936=AXIS2_PLACEMENT_3D('',#19287,#15390,#15391);
#12937=AXIS2_PLACEMENT_3D('',#19288,#15392,#15393);
#12938=AXIS2_PLACEMENT_3D('',#19289,#15394,#15395);
#12939=AXIS2_PLACEMENT_3D('',#19290,#15396,#15397);
#12940=AXIS2_PLACEMENT_3D('',#19291,#15398,#15399);
#12941=AXIS2_PLACEMENT_3D('',#19292,#15400,#15401);
#12942=AXIS2_PLACEMENT_3D('',#19293,#15402,#15403);
#12943=AXIS2_PLACEMENT_3D('',#19294,#15404,#15405);
#15173=DIRECTION('axis',(0.,0.,1.));
#15174=DIRECTION('refdir',(1.,0.,0.));
#15175=DIRECTION('center_axis',(-0.0498412966806705,0.998757150234825,-3.03153484454085E-17));
#15176=DIRECTION('ref_axis',(-1.51095627584551E-18,3.02776710217119E-17,
1.));
#15177=DIRECTION('center_axis',(-0.0498412966806705,0.998757150234825,-3.03153484454085E-17));
#15178=DIRECTION('ref_axis',(1.51095627584551E-18,-3.02776710217119E-17,
-1.));
#15179=DIRECTION('',(-0.0352431188660326,0.706227953689593,-0.707106781186551));
#15180=DIRECTION('center_axis',(0.0498412966806705,-0.998757150234825,3.03153484454085E-17));
#15181=DIRECTION('ref_axis',(1.51095627584551E-18,-3.02776710217119E-17,
-1.));
#15182=DIRECTION('center_axis',(-8.1583057089881E-17,-6.47172530465054E-17,
-1.));
#15183=DIRECTION('ref_axis',(-0.0498412966806691,0.998757150234825,0.));
#15184=DIRECTION('center_axis',(-8.1583057089881E-17,-6.47172530465054E-17,
-1.));
#15185=DIRECTION('ref_axis',(-0.0498412966806713,0.998757150234825,-6.05706138712209E-17));
#15186=DIRECTION('center_axis',(0.998757150234825,0.0498412966806704,-8.47072534159835E-17));
#15187=DIRECTION('ref_axis',(0.0498412966806704,-0.998757150234825,0.));
#15188=DIRECTION('center_axis',(8.1583057089881E-17,6.47172530465054E-17,
1.));
#15189=DIRECTION('ref_axis',(-0.0498412966806706,0.998757150234825,-6.05706138712209E-17));
#15190=DIRECTION('center_axis',(8.1583057089881E-17,6.47172530465054E-17,
1.));
#15191=DIRECTION('ref_axis',(-0.0498412966806706,0.998757150234825,-6.05706138712209E-17));
#15192=DIRECTION('center_axis',(9.07647421261732E-17,-1.19272213358314E-16,
1.));
#15193=DIRECTION('ref_axis',(0.0498412966806691,-0.998757150234825,0.));
#15194=DIRECTION('center_axis',(9.07647421261732E-17,-1.19272213358314E-16,
1.));
#15195=DIRECTION('ref_axis',(0.0498412966806713,-0.998757150234825,-1.23647808356405E-16));
#15196=DIRECTION('center_axis',(0.998757150234825,0.0498412966806703,-8.47072534159836E-17));
#15197=DIRECTION('ref_axis',(-0.0498412966806703,0.998757150234825,0.));
#15198=DIRECTION('center_axis',(-9.07647421261732E-17,1.19272213358314E-16,
-1.));
#15199=DIRECTION('ref_axis',(0.0498412966806706,-0.998757150234825,-1.23647808356405E-16));
#15200=DIRECTION('center_axis',(-9.07647421261732E-17,1.19272213358314E-16,
-1.));
#15201=DIRECTION('ref_axis',(0.0498412966806706,-0.998757150234825,-1.23647808356405E-16));
#15202=DIRECTION('center_axis',(-8.31133379292631E-17,-3.40523419790356E-17,
-1.));
#15203=DIRECTION('ref_axis',(-0.998757150234825,-0.0498412966806706,8.47072534159836E-17));
#15204=DIRECTION('',(8.31133379292631E-17,3.40523419790356E-17,1.));
#15205=DIRECTION('center_axis',(-0.0498412966806705,0.998757150234825,-1.14936005810131E-16));
#15206=DIRECTION('ref_axis',(-5.728559564874E-18,1.147931576223E-16,1.));
#15207=DIRECTION('center_axis',(0.0498412966806705,-0.998757150234825,1.14936005810131E-16));
#15208=DIRECTION('ref_axis',(5.728559564874E-18,-1.147931576223E-16,-1.));
#15209=DIRECTION('',(-0.0498412966806705,0.998757150234825,-1.14936005810131E-16));
#15210=DIRECTION('center_axis',(0.0498412966806705,-0.998757150234825,1.14936005810131E-16));
#15211=DIRECTION('ref_axis',(5.728559564874E-18,-1.147931576223E-16,-1.));
#15212=DIRECTION('center_axis',(-0.0498412966806705,0.998757150234825,-1.14936005810131E-16));
#15213=DIRECTION('ref_axis',(-5.728559564874E-18,1.147931576223E-16,1.));
#15214=DIRECTION('center_axis',(0.0498412966806705,-0.998757150234825,1.14936005810131E-16));
#15215=DIRECTION('ref_axis',(5.728559564874E-18,-1.147931576223E-16,-1.));
#15216=DIRECTION('',(0.0498412966806705,-0.998757150234825,1.14936005810131E-16));
#15217=DIRECTION('center_axis',(0.0498412966806705,-0.998757150234825,1.14936005810131E-16));
#15218=DIRECTION('ref_axis',(5.728559564874E-18,-1.147931576223E-16,-1.));
#15219=DIRECTION('center_axis',(0.0498412966806705,-0.998757150234825,1.14936005810131E-16));
#15220=DIRECTION('ref_axis',(5.728559564874E-18,-1.147931576223E-16,-1.));
#15221=DIRECTION('center_axis',(-0.0498412966806705,0.998757150234825,-3.03153484454085E-17));
#15222=DIRECTION('ref_axis',(-1.51095627584551E-18,3.02776710217119E-17,
1.));
#15223=DIRECTION('center_axis',(0.0498412966806705,-0.998757150234825,-1.57222324633165E-16));
#15224=DIRECTION('ref_axis',(7.83616452686627E-18,-1.57026920903915E-16,
1.));
#15225=DIRECTION('',(-0.0498412966806705,0.998757150234825,-3.03153484454085E-17));
#15226=DIRECTION('center_axis',(0.0498412966806705,-0.998757150234825,3.03153484454085E-17));
#15227=DIRECTION('ref_axis',(1.51095627584551E-18,-3.02776710217119E-17,
-1.));
#15228=DIRECTION('center_axis',(-0.0498412966806705,0.998757150234825,-3.03153484454085E-17));
#15229=DIRECTION('ref_axis',(-1.51095627584551E-18,3.02776710217119E-17,
1.));
#15230=DIRECTION('center_axis',(-0.0498412966806705,0.998757150234825,8.16022951659984E-17));
#15231=DIRECTION('ref_axis',(4.06716420319217E-18,-8.15008757726136E-17,
1.));
#15232=DIRECTION('',(-0.0498412966806705,0.998757150234825,-3.03153484454085E-17));
#15233=DIRECTION('center_axis',(-8.31133379292631E-17,-3.40523419790356E-17,
-1.));
#15234=DIRECTION('ref_axis',(-0.998757150234825,-0.0498412966806714,8.47072534159836E-17));
#15235=DIRECTION('center_axis',(8.31133379292631E-17,3.40523419790356E-17,
1.));
#15236=DIRECTION('ref_axis',(0.998757150234825,0.0498412966806714,-8.47072534159836E-17));
#15237=DIRECTION('',(-8.31133379292631E-17,-3.40523419790356E-17,-1.));
#15238=DIRECTION('center_axis',(8.31133379292631E-17,3.40523419790356E-17,
1.));
#15239=DIRECTION('ref_axis',(0.998757150234825,0.0498412966806714,-8.47072534159836E-17));
#15240=DIRECTION('center_axis',(-8.31133379292631E-17,-3.40523419790356E-17,
-1.));
#15241=DIRECTION('ref_axis',(-0.998757150234825,-0.0498412966806714,8.47072534159836E-17));
#15242=DIRECTION('center_axis',(8.31133379292631E-17,3.40523419790356E-17,
1.));
#15243=DIRECTION('ref_axis',(0.998757150234825,0.0498412966806714,-8.47072534159836E-17));
#15244=DIRECTION('',(-8.31133379292631E-17,-3.40523419790356E-17,-1.));
#15245=DIRECTION('center_axis',(9.07647421261732E-17,-1.19272213358314E-16,
1.));
#15246=DIRECTION('ref_axis',(0.049841296680668,-0.998757150234825,-1.23647808356404E-16));
#15247=DIRECTION('center_axis',(-8.31133379292631E-17,-3.40523419790356E-17,
-1.));
#15248=DIRECTION('ref_axis',(-0.998757150234825,-0.0498412966806712,8.47072534159835E-17));
#15249=DIRECTION('center_axis',(-8.1583057089881E-17,-6.47172530465054E-17,
-1.));
#15250=DIRECTION('ref_axis',(-0.0498412966806713,0.998757150234825,-6.05706138712209E-17));
#15251=DIRECTION('',(-8.31133379292631E-17,-3.40523419790356E-17,-1.));
#15252=DIRECTION('center_axis',(8.31133379292631E-17,3.40523419790356E-17,
1.));
#15253=DIRECTION('ref_axis',(0.998757150234825,0.0498412966806713,-8.47072534159836E-17));
#15254=DIRECTION('',(-8.31133379292631E-17,-3.40523419790356E-17,-1.));
#15255=DIRECTION('center_axis',(-8.31133379292631E-17,-3.40523419790356E-17,
-1.));
#15256=DIRECTION('ref_axis',(-0.998757150234825,-0.0498412966806714,8.47072534159836E-17));
#15257=DIRECTION('center_axis',(-8.1583057089881E-17,-6.47172530465054E-17,
-1.));
#15258=DIRECTION('ref_axis',(-0.0498412966806681,0.998757150234825,-6.05706138712212E-17));
#15259=DIRECTION('',(-8.31133379292631E-17,-3.40523419790356E-17,-1.));
#15260=DIRECTION('center_axis',(8.31133379292631E-17,3.40523419790356E-17,
1.));
#15261=DIRECTION('ref_axis',(0.998757150234825,0.0498412966806714,-8.47072534159836E-17));
#15262=DIRECTION('center_axis',(-8.31133379292631E-17,-3.40523419790356E-17,
-1.));
#15263=DIRECTION('ref_axis',(-0.998757150234825,-0.0498412966806712,8.47072534159835E-17));
#15264=DIRECTION('center_axis',(8.31133379292631E-17,3.40523419790356E-17,
1.));
#15265=DIRECTION('ref_axis',(0.998757150234825,0.0498412966806713,-8.47072534159836E-17));
#15266=DIRECTION('',(-8.31133379292631E-17,-3.40523419790356E-17,-1.));
#15267=DIRECTION('center_axis',(9.07647421261732E-17,-1.19272213358314E-16,
1.));
#15268=DIRECTION('ref_axis',(0.0498412966806712,-0.998757150234825,-1.23647808356405E-16));
#15269=DIRECTION('',(-8.31133379292631E-17,-3.40523419790356E-17,-1.));
#15270=DIRECTION('center_axis',(0.998757150234825,0.0498412966806707,-7.55063512648625E-17));
#15271=DIRECTION('ref_axis',(-7.54125082139238E-17,-3.76333445466695E-18,
-1.));
#15272=DIRECTION('',(0.998757150234825,0.0498412966806707,-7.55063512648625E-17));
#15273=DIRECTION('center_axis',(0.998757150234825,0.0498412966806707,-7.55063512648625E-17));
#15274=DIRECTION('ref_axis',(-7.54125082139238E-17,-3.76333445466695E-18,
-1.));
#15275=DIRECTION('',(0.998757150234825,0.0498412966806707,-7.55063512648625E-17));
#15276=DIRECTION('center_axis',(0.998757150234825,0.0498412966806708,-7.55063512648625E-17));
#15277=DIRECTION('ref_axis',(-0.0498412966806708,0.998757150234825,-3.22015486701546E-31));
#15278=DIRECTION('',(0.998757150234825,0.0498412966806707,-7.55063512648625E-17));
#15279=DIRECTION('center_axis',(-0.0498412966806705,0.998757150234825,8.20501001114569E-17));
#15280=DIRECTION('ref_axis',(8.86914584083007E-17,-7.772620481529E-17,1.));
#15281=DIRECTION('',(8.86914584083008E-17,-7.772620481529E-17,1.));
#15282=DIRECTION('',(0.998757150234825,0.0498412966806707,-7.55063512648625E-17));
#15283=DIRECTION('center_axis',(0.998757150234825,0.0498412966806707,-7.55063512648625E-17));
#15284=DIRECTION('ref_axis',(-7.54125082139238E-17,-3.76333445466695E-18,
-1.));
#15285=DIRECTION('center_axis',(0.998757150234825,0.0498412966806708,-7.55063512648625E-17));
#15286=DIRECTION('ref_axis',(-0.0498412966806708,0.998757150234825,-3.22015486701546E-31));
#15287=DIRECTION('',(0.998757150234825,0.0498412966806707,-7.55063512648625E-17));
#15288=DIRECTION('center_axis',(0.998757150234825,0.0498412966806707,-7.55063512648625E-17));
#15289=DIRECTION('ref_axis',(-7.54125082139238E-17,-3.76333445466695E-18,
-1.));
#15290=DIRECTION('',(0.998757150234825,0.0498412966806707,-7.55063512648625E-17));
#15291=DIRECTION('center_axis',(0.962724230937995,-0.270484852006255,-6.19392384262883E-17));
#15292=DIRECTION('ref_axis',(0.270484852006255,0.962724230937995,-5.27613511566066E-17));
#15293=DIRECTION('',(0.270484852006255,0.962724230937995,-8.18692862944502E-17));
#15294=DIRECTION('',(-8.31133379292631E-17,-3.40523419790356E-17,-1.));
#15295=DIRECTION('',(-0.270484852006255,-0.962724230937995,5.27613511566066E-17));
#15296=DIRECTION('center_axis',(-0.73203038565962,0.68127198274333,3.09069982706067E-17));
#15297=DIRECTION('ref_axis',(-0.68127198274333,-0.73203038565962,7.52661071837786E-17));
#15298=DIRECTION('',(0.68127198274333,0.73203038565962,-7.52661071837786E-17));
#15299=DIRECTION('',(8.31133379292631E-17,3.40523419790356E-17,1.));
#15300=DIRECTION('',(-0.68127198274333,-0.73203038565962,9.66712163971166E-17));
#15301=DIRECTION('center_axis',(7.39238711172199E-17,3.35937570851917E-17,
1.));
#15302=DIRECTION('ref_axis',(0.998757150234825,0.0498412966806707,-7.55063512648625E-17));
#15303=DIRECTION('',(0.68127198274333,0.73203038565962,-7.52661071837786E-17));
#15304=DIRECTION('center_axis',(8.31133379292631E-17,3.40523419790356E-17,
1.));
#15305=DIRECTION('ref_axis',(0.998757150234825,0.0498412966806708,-8.47072534159836E-17));
#15306=DIRECTION('',(-0.0498412966806705,0.998757150234825,-3.03153484454085E-17));
#15307=DIRECTION('',(-0.998757150234825,-0.0498412966806707,7.55063512648625E-17));
#15308=DIRECTION('',(0.0498412966806706,-0.998757150234825,3.03153484454085E-17));
#15309=DIRECTION('center_axis',(-8.31133379292631E-17,-3.40523419790356E-17,
-1.));
#15310=DIRECTION('ref_axis',(0.998757150234825,0.0498412966806708,-8.47072534159836E-17));
#15311=DIRECTION('',(-0.270484852006255,-0.962724230937995,5.27613511566066E-17));
#15312=DIRECTION('center_axis',(7.39238711172199E-17,3.35937570851917E-17,
1.));
#15313=DIRECTION('ref_axis',(0.998757150234825,0.0498412966806707,-7.55063512648625E-17));
#15314=DIRECTION('',(-0.0498412966806705,0.998757150234825,-3.03153484454085E-17));
#15315=DIRECTION('center_axis',(-8.31133379292631E-17,-3.40523419790356E-17,
-1.));
#15316=DIRECTION('ref_axis',(0.998757150234825,0.0498412966806708,-8.47072534159836E-17));
#15317=DIRECTION('center_axis',(8.31133379292631E-17,3.40523419790356E-17,
1.));
#15318=DIRECTION('ref_axis',(0.998757150234825,0.0498412966806708,-8.47072534159836E-17));
#15319=DIRECTION('',(0.0498412966806706,-0.998757150234825,3.03153484454085E-17));
#15320=DIRECTION('',(0.998757150234825,0.0498412966806707,-7.55063512648625E-17));
#15321=DIRECTION('center_axis',(0.0498412966806705,-0.998757150234825,2.986754349995E-17));
#15322=DIRECTION('ref_axis',(-8.31133379292631E-17,-3.40523419790355E-17,
-1.));
#15323=DIRECTION('',(-8.31133379292631E-17,-3.40523419790356E-17,-1.));
#15324=DIRECTION('',(-0.998757150234825,-0.0498412966806707,7.55063512648625E-17));
#15325=DIRECTION('',(-8.31133379292631E-17,-3.40523419790356E-17,-1.));
#15326=DIRECTION('',(0.998757150234825,0.0498412966806707,-7.55063512648625E-17));
#15327=DIRECTION('center_axis',(0.998757150234825,0.0498412966806706,-7.55063512648625E-17));
#15328=DIRECTION('ref_axis',(-0.0498412966806706,0.998757150234825,-3.03153484454085E-17));
#15329=DIRECTION('',(0.0498412966806706,-0.998757150234825,-1.23200003410946E-16));
#15330=DIRECTION('',(8.31133379292631E-17,3.40523419790356E-17,1.));
#15331=DIRECTION('center_axis',(-0.998757150234825,-0.0498412966806708,
7.55063512648625E-17));
#15332=DIRECTION('ref_axis',(-0.0498412966806708,0.998757150234825,2.19556013660145E-31));
#15333=DIRECTION('center_axis',(-0.998757150234825,-0.0498412966806708,
7.55063512648625E-17));
#15334=DIRECTION('ref_axis',(-0.0498412966806708,0.998757150234825,2.19556013660145E-31));
#15335=DIRECTION('',(8.31133379292631E-17,3.40523419790356E-17,1.));
#15336=DIRECTION('',(-0.0498412966806706,0.998757150234825,-6.10184188166794E-17));
#15337=DIRECTION('',(9.24604587319749E-17,-1.53252249946591E-16,1.));
#15338=DIRECTION('',(0.0498412966806706,-0.998757150234825,-1.43156999152272E-16));
#15339=DIRECTION('',(-8.31133379292631E-17,-3.40523419790356E-17,-1.));
#15340=DIRECTION('',(-0.0498412966806706,0.998757150234825,-3.03153484454085E-17));
#15341=DIRECTION('center_axis',(0.962724230937995,-0.270484852006255,-6.19392384262883E-17));
#15342=DIRECTION('ref_axis',(0.270484852006255,0.962724230937995,-5.27613511566066E-17));
#15343=DIRECTION('',(-8.31133379292631E-17,-3.40523419790356E-17,-1.));
#15344=DIRECTION('',(-0.270484852006255,-0.962724230937995,-9.27783245326118E-17));
#15345=DIRECTION('center_axis',(-0.73203038565962,0.68127198274333,3.09069982706067E-17));
#15346=DIRECTION('ref_axis',(-0.68127198274333,-0.73203038565962,7.52661071837786E-17));
#15347=DIRECTION('',(0.68127198274333,0.73203038565962,3.17594388829113E-17));
#15348=DIRECTION('',(8.31133379292631E-17,3.40523419790356E-17,1.));
#15349=DIRECTION('center_axis',(-0.998757150234825,-0.0498412966806707,
8.47072534159836E-17));
#15350=DIRECTION('ref_axis',(8.31133379292631E-17,3.40523419790356E-17,
1.));
#15351=DIRECTION('',(-0.0498412966806705,0.998757150234825,-6.10184188166794E-17));
#15352=DIRECTION('',(-8.31133379292631E-17,-3.40523419790356E-17,-1.));
#15353=DIRECTION('center_axis',(0.998757150234825,0.0498412966806707,-7.55063512648625E-17));
#15354=DIRECTION('ref_axis',(7.54125082139238E-17,3.76333445466695E-18,
1.));
#15355=DIRECTION('center_axis',(0.998757150234825,0.0498412966806707,-7.55063512648625E-17));
#15356=DIRECTION('ref_axis',(7.54125082139238E-17,3.76333445466695E-18,
1.));
#15357=DIRECTION('',(-8.31133379292631E-17,-3.40523419790356E-17,-1.));
#15358=DIRECTION('',(0.0498412966806705,-0.998757150234825,-1.23200003410946E-16));
#15359=DIRECTION('',(9.24604587319749E-17,-1.53252249946591E-16,1.));
#15360=DIRECTION('',(-0.0498412966806705,0.998757150234825,-3.03153484454085E-17));
#15361=DIRECTION('',(-8.31133379292631E-17,-3.40523419790356E-17,-1.));
#15362=DIRECTION('',(0.0498412966806705,-0.998757150234825,-1.43156999152272E-16));
#15363=DIRECTION('',(8.86914584083008E-17,-7.772620481529E-17,1.));
#15364=DIRECTION('center_axis',(-0.998757150234825,-0.0498412966806707,
7.55063512648625E-17));
#15365=DIRECTION('ref_axis',(7.54125082139238E-17,3.76333445466695E-18,
1.));
#15366=DIRECTION('center_axis',(0.998757150234825,0.0498412966806707,-7.55063512648625E-17));
#15367=DIRECTION('ref_axis',(-7.54125082139238E-17,-3.76333445466695E-18,
-1.));
#15368=DIRECTION('center_axis',(-0.0498412966806705,0.998757150234825,1.57670129578624E-16));
#15369=DIRECTION('ref_axis',(9.24604587319748E-17,-1.53252249946591E-16,
1.));
#15370=DIRECTION('',(0.998757150234825,0.0498412966806707,-7.55063512648625E-17));
#15371=DIRECTION('',(0.998757150234825,0.0498412966806707,-7.55063512648625E-17));
#15372=DIRECTION('center_axis',(-8.15607379107394E-17,-6.51645014376925E-17,
-1.));
#15373=DIRECTION('ref_axis',(-0.0498412966806705,0.998757150234825,-6.10184188166794E-17));
#15374=DIRECTION('center_axis',(8.1583057089881E-17,6.47172530465054E-17,
1.));
#15375=DIRECTION('ref_axis',(-0.0498412966806736,0.998757150234825,-6.05706138712207E-17));
#15376=DIRECTION('center_axis',(-8.1583057089881E-17,-6.47172530465054E-17,
-1.));
#15377=DIRECTION('ref_axis',(-0.0498412966806694,0.998757150234825,-6.05706138712211E-17));
#15378=DIRECTION('center_axis',(9.07424229470315E-17,-1.18824964967127E-16,
1.));
#15379=DIRECTION('ref_axis',(0.0498412966806705,-0.998757150234825,-1.23200003410946E-16));
#15380=DIRECTION('center_axis',(-9.07647421261732E-17,1.19272213358314E-16,
-1.));
#15381=DIRECTION('ref_axis',(0.0498412966806736,-0.998757150234825,-1.23647808356405E-16));
#15382=DIRECTION('center_axis',(9.07647421261732E-17,-1.19272213358314E-16,
1.));
#15383=DIRECTION('ref_axis',(0.0498412966806694,-0.998757150234825,-1.23647808356405E-16));
#15384=DIRECTION('center_axis',(0.0498412966806705,-0.998757150234825,2.986754349995E-17));
#15385=DIRECTION('ref_axis',(-8.31133379292631E-17,-3.40523419790355E-17,
-1.));
#15386=DIRECTION('',(0.998757150234825,0.0498412966806707,-7.55063512648625E-17));
#15387=DIRECTION('',(0.998757150234825,0.0498412966806707,-7.55063512648625E-17));
#15388=DIRECTION('center_axis',(9.17371054926298E-17,-1.38757157160982E-16,
1.));
#15389=DIRECTION('ref_axis',(0.0498412966806705,-0.998757150234825,-1.43156999152272E-16));
#15390=DIRECTION('center_axis',(-0.0498412966806705,0.998757150234825,8.20501001114569E-17));
#15391=DIRECTION('ref_axis',(8.86914584083007E-17,-7.772620481529E-17,1.));
#15392=DIRECTION('center_axis',(-7.39238711172199E-17,-3.35937570851917E-17,
-1.));
#15393=DIRECTION('ref_axis',(-0.998757150234825,-0.0498412966806707,7.55063512648625E-17));
#15394=DIRECTION('center_axis',(0.0498412966806705,-0.998757150234825,1.14488200864672E-16));
#15395=DIRECTION('ref_axis',(-7.88957346402346E-17,-1.18567828579623E-16,
-1.));
#15396=DIRECTION('center_axis',(0.0498412966806705,-0.998757150234825,1.14488200864672E-16));
#15397=DIRECTION('ref_axis',(-7.88957346402346E-17,-1.18567828579623E-16,
-1.));
#15398=DIRECTION('center_axis',(8.31133379292631E-17,3.40523419790356E-17,
1.));
#15399=DIRECTION('ref_axis',(0.998757150234825,0.0498412966806708,-8.47072534159836E-17));
#15400=DIRECTION('center_axis',(8.31133379292631E-17,3.40523419790356E-17,
1.));
#15401=DIRECTION('ref_axis',(0.998757150234825,0.0498412966806708,-8.47072534159836E-17));
#15402=DIRECTION('center_axis',(-8.31133379292631E-17,-3.40523419790356E-17,
-1.));
#15403=DIRECTION('ref_axis',(-0.998757150234825,-0.0498412966806708,8.47072534159836E-17));
#15404=DIRECTION('center_axis',(-8.31133379292631E-17,-3.40523419790356E-17,
-1.));
#15405=DIRECTION('ref_axis',(-0.998757150234825,-0.0498412966806708,8.47072534159836E-17));
#19044=CARTESIAN_POINT('',(0.,0.,0.));
#19045=CARTESIAN_POINT('Origin',(-235.27780721626,263.259715347801,253.073593133701));
#19046=CARTESIAN_POINT('',(-235.27780721626,263.259715347801,239.573593133701));
#19047=CARTESIAN_POINT('Origin',(-235.27780721626,263.259715347801,253.073593133701));
#19048=CARTESIAN_POINT('',(-235.327648512941,264.258472498036,238.573593133701));
#19049=CARTESIAN_POINT('',(-235.27780721626,263.259715347801,239.573593133701));
#19050=CARTESIAN_POINT('Origin',(-235.327648512941,264.258472498036,253.073593133701));
#19051=CARTESIAN_POINT('Origin',(-232.939627118478,176.278148255512,236.573593133701));
#19052=CARTESIAN_POINT('',(-232.192007668268,161.29679100199,234.573593133701));
#19053=CARTESIAN_POINT('Origin',(-232.939627118478,176.278148255512,234.573593133701));
#19054=CARTESIAN_POINT('',(-232.29169026163,163.29430530246,236.573593133701));
#19055=CARTESIAN_POINT('Origin',(-232.192007668268,161.29679100199,236.573593133701));
#19056=CARTESIAN_POINT('',(-219.955784165426,176.926085112361,236.573593133701));
#19057=CARTESIAN_POINT('Origin',(-232.939627118478,176.278148255512,236.573593133701));
#19058=CARTESIAN_POINT('Origin',(-232.939627118478,176.278148255512,236.573593133701));
#19059=CARTESIAN_POINT('Origin',(-232.939627118478,176.278148255512,269.573593133701));
#19060=CARTESIAN_POINT('',(-233.687246568689,191.259505509035,271.573593133701));
#19061=CARTESIAN_POINT('Origin',(-232.939627118478,176.278148255512,271.573593133701));
#19062=CARTESIAN_POINT('',(-233.587563975327,189.261991208565,269.573593133701));
#19063=CARTESIAN_POINT('Origin',(-233.687246568688,191.259505509035,269.573593133701));
#19064=CARTESIAN_POINT('',(-219.955784165426,176.926085112361,269.573593133701));
#19065=CARTESIAN_POINT('Origin',(-232.939627118478,176.278148255512,269.573593133701));
#19066=CARTESIAN_POINT('Origin',(-232.939627118478,176.278148255512,269.573593133701));
#19067=CARTESIAN_POINT('Origin',(-232.939627118478,176.278148255512,276.575593133701));
#19068=CARTESIAN_POINT('',(-219.955784165426,176.926085112361,276.575593133701));
#19069=CARTESIAN_POINT('Origin',(-234.829235546134,254.270900995688,253.073593133701));
#19070=CARTESIAN_POINT('',(-234.829235546134,254.270900995688,240.573593133701));
#19071=CARTESIAN_POINT('Origin',(-234.829235546134,254.270900995688,253.073593133701));
#19072=CARTESIAN_POINT('',(-235.078442029538,259.264686746862,240.573593133701));
#19073=CARTESIAN_POINT('',(-234.829235546134,254.270900995688,240.573593133701));
#19074=CARTESIAN_POINT('Origin',(-235.078442029538,259.264686746862,253.073593133701));
#19075=CARTESIAN_POINT('Origin',(-234.829235546134,254.270900995688,253.073593133701));
#19076=CARTESIAN_POINT('',(-225.938313363545,259.720809503464,268.573593133701));
#19077=CARTESIAN_POINT('',(-244.218570695531,258.80856399026,268.573593133701));
#19078=CARTESIAN_POINT('Ctrl Pts',(-244.218570695531,258.80856399026,268.573593133701));
#19079=CARTESIAN_POINT('Ctrl Pts',(-243.882569447187,258.825331567743,268.772221695988));
#19080=CARTESIAN_POINT('Ctrl Pts',(-243.537504054999,258.822928410752,268.960846032026));
#19081=CARTESIAN_POINT('Ctrl Pts',(-242.350109030347,258.767377256699,269.558780483369));
#19082=CARTESIAN_POINT('Ctrl Pts',(-241.471668538286,258.64932649441,269.917592682587));
#19083=CARTESIAN_POINT('Ctrl Pts',(-238.761208602761,258.222554255849,270.783055750245));
#19084=CARTESIAN_POINT('Ctrl Pts',(-236.856253783888,257.832610843749,271.073593133701));
#19085=CARTESIAN_POINT('Ctrl Pts',(-233.166887375258,258.01672247258,271.073593133701));
#19086=CARTESIAN_POINT('Ctrl Pts',(-231.310219222211,258.594383355839,270.783055750245));
#19087=CARTESIAN_POINT('Ctrl Pts',(-228.655714581594,259.288885133116,269.917592682587));
#19088=CARTESIAN_POINT('Ctrl Pts',(-227.793391434726,259.493805778597,269.558780483369));
#19089=CARTESIAN_POINT('Ctrl Pts',(-226.617426357145,259.667296445764,268.960846032026));
#19090=CARTESIAN_POINT('Ctrl Pts',(-226.274314611889,259.704041925981,268.772221695988));
#19091=CARTESIAN_POINT('Ctrl Pts',(-225.938313363545,259.720809503464,268.573593133701));
#19092=CARTESIAN_POINT('',(-244.218570695531,258.80856399026,237.573593133701));
#19093=CARTESIAN_POINT('Origin',(-235.078442029538,259.264686746862,253.073593133701));
#19094=CARTESIAN_POINT('',(-235.011570579573,257.924666658164,235.073593133701));
#19095=CARTESIAN_POINT('Ctrl Pts',(-244.218570695531,258.80856399026,237.573593133701));
#19096=CARTESIAN_POINT('Ctrl Pts',(-243.882569447187,258.825331567743,237.374964571413));
#19097=CARTESIAN_POINT('Ctrl Pts',(-243.537504054999,258.822928410752,237.186340235375));
#19098=CARTESIAN_POINT('Ctrl Pts',(-242.350109030347,258.767377256699,236.588405784032));
#19099=CARTESIAN_POINT('Ctrl Pts',(-241.471668538286,258.64932649441,236.229593584814));
#19100=CARTESIAN_POINT('Ctrl Pts',(-238.761208602761,258.222554255849,235.364130517157));
#19101=CARTESIAN_POINT('Ctrl Pts',(-236.856253783888,257.832610843749,235.073593133701));
#19102=CARTESIAN_POINT('Ctrl Pts',(-235.011570579573,257.924666658164,235.073593133701));
#19103=CARTESIAN_POINT('',(-234.829235546134,254.270900995688,235.073593133701));
#19104=CARTESIAN_POINT('',(-234.829235546134,254.270900995688,235.073593133701));
#19105=CARTESIAN_POINT('Origin',(-234.829235546134,254.270900995688,253.073593133701));
#19106=CARTESIAN_POINT('',(-225.938313363544,259.720809503464,237.573593133701));
#19107=CARTESIAN_POINT('Ctrl Pts',(-235.011570579573,257.924666658164,235.073593133701));
#19108=CARTESIAN_POINT('Ctrl Pts',(-233.166887375258,258.01672247258,235.073593133701));
#19109=CARTESIAN_POINT('Ctrl Pts',(-231.310219222211,258.594383355839,235.364130517156));
#19110=CARTESIAN_POINT('Ctrl Pts',(-228.655714581594,259.288885133116,236.229593584814));
#19111=CARTESIAN_POINT('Ctrl Pts',(-227.793391434726,259.493805778597,236.588405784032));
#19112=CARTESIAN_POINT('Ctrl Pts',(-226.617426357145,259.667296445764,237.186340235375));
#19113=CARTESIAN_POINT('Ctrl Pts',(-226.274314611889,259.704041925981,237.374964571413));
#19114=CARTESIAN_POINT('Ctrl Pts',(-225.938313363545,259.720809503464,237.573593133701));
#19115=CARTESIAN_POINT('Origin',(-235.078442029538,259.264686746862,253.073593133701));
#19116=CARTESIAN_POINT('Origin',(-231.779757303713,193.163177041049,253.073593133701));
#19117=CARTESIAN_POINT('',(-233.682885722479,231.299486540287,239.573593133701));
#19118=CARTESIAN_POINT('Origin',(-233.682885722479,231.299486540287,253.073593133701));
#19119=CARTESIAN_POINT('',(-233.932092205882,236.293272291461,239.573593133701));
#19120=CARTESIAN_POINT('',(-231.779757303713,193.163177041049,239.573593133701));
#19121=CARTESIAN_POINT('Origin',(-233.932092205882,236.293272291461,253.073593133701));
#19122=CARTESIAN_POINT('Origin',(-231.779757303713,193.163177041049,253.073593133701));
#19123=CARTESIAN_POINT('',(-235.078442029538,259.264686746862,239.573593133701));
#19124=CARTESIAN_POINT('Origin',(-235.078442029538,259.264686746862,253.073593133701));
#19125=CARTESIAN_POINT('',(-231.779757303713,193.163177041049,239.573593133701));
#19126=CARTESIAN_POINT('Origin',(-232.939627118478,176.278148255512,276.573593133701));
#19127=CARTESIAN_POINT('',(-224.9495699166,176.676878628958,276.573593133701));
#19128=CARTESIAN_POINT('Origin',(-232.939627118478,176.278148255512,276.573593133701));
#19129=CARTESIAN_POINT('',(-224.9495699166,176.676878628958,229.573593133701));
#19130=CARTESIAN_POINT('',(-224.9495699166,176.676878628958,276.573593133701));
#19131=CARTESIAN_POINT('Origin',(-232.939627118478,176.278148255512,229.573593133701));
#19132=CARTESIAN_POINT('Origin',(-256.262104047518,132.050757761675,276.573593133701));
#19133=CARTESIAN_POINT('',(-248.272046845639,132.44948813512,276.573593133701));
#19134=CARTESIAN_POINT('Origin',(-256.262104047518,132.050757761675,276.573593133701));
#19135=CARTESIAN_POINT('',(-248.272046845639,132.44948813512,271.573593133701));
#19136=CARTESIAN_POINT('',(-248.272046845639,132.44948813512,276.573593133701));
#19137=CARTESIAN_POINT('Origin',(-256.262104047518,132.050757761675,271.573593133701));
#19138=CARTESIAN_POINT('Origin',(-256.262104047518,132.050757761675,276.573593133701));
#19139=CARTESIAN_POINT('',(-245.281648262624,121.831678020525,234.573593133701));
#19140=CARTESIAN_POINT('',(-270.702967511588,136.108030541768,234.573593133701));
#19141=CARTESIAN_POINT('Origin',(-256.262104047518,132.050757761675,234.573593133701));
#19142=CARTESIAN_POINT('',(-270.702967511588,136.108030541768,229.573593133701));
#19143=CARTESIAN_POINT('',(-270.702967511588,136.108030541768,276.573593133701));
#19144=CARTESIAN_POINT('',(-245.281648262624,121.831678020525,229.573593133701));
#19145=CARTESIAN_POINT('Origin',(-256.262104047518,132.050757761675,229.573593133701));
#19146=CARTESIAN_POINT('',(-245.281648262624,121.831678020525,276.573593133701));
#19147=CARTESIAN_POINT('Origin',(-256.262104047518,132.050757761675,276.573593133701));
#19148=CARTESIAN_POINT('',(-248.272046845639,132.44948813512,234.573593133701));
#19149=CARTESIAN_POINT('Origin',(-256.262104047518,132.050757761675,234.573593133701));
#19150=CARTESIAN_POINT('',(-248.272046845639,132.44948813512,229.573593133701));
#19151=CARTESIAN_POINT('',(-248.272046845639,132.44948813512,276.573593133701));
#19152=CARTESIAN_POINT('Origin',(-256.262104047518,132.050757761675,229.573593133701));
#19153=CARTESIAN_POINT('Origin',(-256.262104047518,132.050757761675,276.573593133701));
#19154=CARTESIAN_POINT('',(-270.702967511588,136.108030541768,276.573593133701));
#19155=CARTESIAN_POINT('',(-245.281648262624,121.831678020525,276.573593133701));
#19156=CARTESIAN_POINT('Origin',(-256.262104047518,132.050757761675,276.573593133701));
#19157=CARTESIAN_POINT('',(-270.702967511588,136.108030541768,271.573593133701));
#19158=CARTESIAN_POINT('',(-270.702967511588,136.108030541768,276.573593133701));
#19159=CARTESIAN_POINT('',(-245.281648262624,121.831678020525,271.573593133701));
#19160=CARTESIAN_POINT('Origin',(-256.262104047518,132.050757761675,271.573593133701));
#19161=CARTESIAN_POINT('',(-245.281648262624,121.831678020525,276.573593133701));
#19162=CARTESIAN_POINT('Origin',(-277.373940792763,254.150267790348,268.573593133701));
#19163=CARTESIAN_POINT('',(-205.115727522493,260.759925647282,268.573593133701));
#19164=CARTESIAN_POINT('',(-277.523464682805,257.146539241052,268.573593133701));
#19165=CARTESIAN_POINT('',(-204.966203632451,257.763654196578,271.573593133701));
#19166=CARTESIAN_POINT('Origin',(-204.966203632451,257.763654196578,268.573593133701));
#19167=CARTESIAN_POINT('',(-264.89163264654,254.773176395737,271.573593133701));
#19168=CARTESIAN_POINT('',(-277.373940792763,254.150267790348,271.573593133701));
#19169=CARTESIAN_POINT('',(-265.041156536582,257.769447846442,268.573593133701));
#19170=CARTESIAN_POINT('Origin',(-264.89163264654,254.773176395737,268.573593133701));
#19171=CARTESIAN_POINT('',(-277.523464682805,257.146539241052,268.573593133701));
#19172=CARTESIAN_POINT('Origin',(-277.523464682805,257.146539241052,237.573593133701));
#19173=CARTESIAN_POINT('',(-265.041156536582,257.769447846442,237.573593133701));
#19174=CARTESIAN_POINT('',(-265.041156536582,257.769447846442,276.573593133701));
#19175=CARTESIAN_POINT('',(-277.523464682805,257.146539241052,237.573593133701));
#19176=CARTESIAN_POINT('Origin',(-277.373940792763,254.150267790348,237.573593133701));
#19177=CARTESIAN_POINT('',(-264.89163264654,254.773176395737,234.573593133701));
#19178=CARTESIAN_POINT('Origin',(-264.89163264654,254.773176395737,237.573593133701));
#19179=CARTESIAN_POINT('',(-204.966203632451,257.763654196578,234.573593133701));
#19180=CARTESIAN_POINT('',(-277.373940792763,254.150267790348,234.573593133701));
#19181=CARTESIAN_POINT('',(-205.115727522493,260.759925647282,237.573593133701));
#19182=CARTESIAN_POINT('Origin',(-204.966203632451,257.763654196578,237.573593133701));
#19183=CARTESIAN_POINT('',(-277.523464682805,257.146539241052,237.573593133701));
#19184=CARTESIAN_POINT('Origin',(-260.739538157925,171.570404093794,276.573593133701));
#19185=CARTESIAN_POINT('',(-261.622986471561,168.425987347309,234.573593133701));
#19186=CARTESIAN_POINT('',(-260.739538157925,171.570404093794,234.573593133701));
#19187=CARTESIAN_POINT('',(-261.622986471561,168.425987347309,229.573593133701));
#19188=CARTESIAN_POINT('',(-261.622986471561,168.425987347309,229.573593133701));
#19189=CARTESIAN_POINT('',(-260.739538157925,171.570404093794,229.573593133701));
#19190=CARTESIAN_POINT('Origin',(-245.281648262624,121.831678020525,276.573593133701));
#19191=CARTESIAN_POINT('',(-206.335336816992,163.679697768471,229.573593133701));
#19192=CARTESIAN_POINT('',(-245.281648262624,121.831678020525,229.573593133701));
#19193=CARTESIAN_POINT('',(-206.335336816992,163.679697768471,234.573593133701));
#19194=CARTESIAN_POINT('',(-206.335336816992,163.679697768471,276.573593133701));
#19195=CARTESIAN_POINT('',(-245.281648262624,121.831678020525,234.573593133701));
#19196=CARTESIAN_POINT('Origin',(-256.262104047518,132.050757761675,276.573593133701));
#19197=CARTESIAN_POINT('',(-206.335336816992,163.679697768471,276.573593133701));
#19198=CARTESIAN_POINT('',(-245.281648262624,121.831678020525,276.573593133701));
#19199=CARTESIAN_POINT('',(-201.000801525488,178.301963356951,276.573593133701));
#19200=CARTESIAN_POINT('Origin',(-220.975944530184,177.305137423337,276.573593133701));
#19201=CARTESIAN_POINT('',(-204.966203632451,257.763654196578,276.573593133701));
#19202=CARTESIAN_POINT('',(-200.579725765336,169.864132597105,276.573593133701));
#19203=CARTESIAN_POINT('',(-264.89163264654,254.773176395737,276.573593133701));
#19204=CARTESIAN_POINT('',(-264.89163264654,254.773176395737,276.573593133701));
#19205=CARTESIAN_POINT('',(-260.902328085625,174.832510321047,276.573593133701));
#19206=CARTESIAN_POINT('',(-265.290363019986,262.763233597616,276.573593133701));
#19207=CARTESIAN_POINT('',(-261.622986471561,168.425987347309,276.573593133701));
#19208=CARTESIAN_POINT('Origin',(-280.877471090321,173.835684387434,276.573593133701));
#19209=CARTESIAN_POINT('',(-260.739538157925,171.570404093794,276.573593133701));
#19210=CARTESIAN_POINT('Origin',(-256.262104047518,132.050757761675,229.573593133701));
#19211=CARTESIAN_POINT('',(-201.000801525488,178.301963356951,229.573593133701));
#19212=CARTESIAN_POINT('',(-204.966203632451,257.763654196578,229.573593133701));
#19213=CARTESIAN_POINT('',(-200.579725765336,169.864132597105,229.573593133701));
#19214=CARTESIAN_POINT('Origin',(-220.975944530184,177.305137423337,229.573593133701));
#19215=CARTESIAN_POINT('',(-260.902328085625,174.832510321047,229.573593133701));
#19216=CARTESIAN_POINT('Origin',(-280.877471090321,173.835684387434,229.573593133701));
#19217=CARTESIAN_POINT('',(-264.89163264654,254.773176395737,229.573593133701));
#19218=CARTESIAN_POINT('',(-265.290363019986,262.763233597616,229.573593133701));
#19219=CARTESIAN_POINT('',(-262.39258353924,254.897887240558,229.573593133701));
#19220=CARTESIAN_POINT('Origin',(-205.364934005896,265.753711398456,276.573593133701));
#19221=CARTESIAN_POINT('',(-205.364934005896,265.753711398456,268.573593133701));
#19222=CARTESIAN_POINT('',(-205.364934005896,265.753711398456,237.573593133701));
#19223=CARTESIAN_POINT('',(-205.364934005896,265.753711398456,276.573593133701));
#19224=CARTESIAN_POINT('',(-265.290363019986,262.763233597616,237.573593133701));
#19225=CARTESIAN_POINT('',(-205.364934005896,265.753711398456,237.573593133701));
#19226=CARTESIAN_POINT('',(-265.290363019986,262.763233597616,268.573593133701));
#19227=CARTESIAN_POINT('',(-265.290363019986,262.763233597616,276.573593133701));
#19228=CARTESIAN_POINT('',(-205.364934005896,265.753711398456,268.573593133701));
#19229=CARTESIAN_POINT('Origin',(-265.290363019986,262.763233597616,276.573593133701));
#19230=CARTESIAN_POINT('',(-263.645600229524,229.804247639867,271.573593133701));
#19231=CARTESIAN_POINT('',(-260.902328085625,174.832510321047,271.573593133701));
#19232=CARTESIAN_POINT('',(-265.290363019986,262.763233597616,271.573593133701));
#19233=CARTESIAN_POINT('',(-260.902328085625,174.832510321047,276.573593133701));
#19234=CARTESIAN_POINT('Origin',(-264.89163264654,254.773176395737,268.573593133701));
#19235=CARTESIAN_POINT('Origin',(-264.89163264654,254.773176395737,237.573593133701));
#19236=CARTESIAN_POINT('',(-260.902328085625,174.832510321047,234.573593133701));
#19237=CARTESIAN_POINT('',(-260.902328085625,174.832510321047,234.573593133701));
#19238=CARTESIAN_POINT('',(-263.645600229524,229.804247639867,234.573593133701));
#19239=CARTESIAN_POINT('',(-265.290363019986,262.763233597616,234.573593133701));
#19240=CARTESIAN_POINT('',(-263.645600229524,229.804247639867,276.573593133701));
#19241=CARTESIAN_POINT('',(-263.894806712927,234.798033391041,271.573593133701));
#19242=CARTESIAN_POINT('',(-265.290363019986,262.763233597616,271.573593133701));
#19243=CARTESIAN_POINT('',(-263.894806712927,234.798033391041,234.573593133701));
#19244=CARTESIAN_POINT('',(-263.894806712927,234.798033391041,276.573593133701));
#19245=CARTESIAN_POINT('',(-265.290363019986,262.763233597616,234.573593133701));
#19246=CARTESIAN_POINT('Origin',(-260.739538157925,171.570404093794,276.573593133701));
#19247=CARTESIAN_POINT('',(-261.622986471561,168.425987347309,271.573593133701));
#19248=CARTESIAN_POINT('',(-261.622986471561,168.425987347309,271.573593133701));
#19249=CARTESIAN_POINT('',(-260.739538157925,171.570404093794,271.573593133701));
#19250=CARTESIAN_POINT('Origin',(-245.281648262624,121.831678020525,276.573593133701));
#19251=CARTESIAN_POINT('',(-206.335336816992,163.679697768471,271.573593133701));
#19252=CARTESIAN_POINT('',(-245.281648262624,121.831678020525,271.573593133701));
#19253=CARTESIAN_POINT('',(-206.335336816992,163.679697768471,276.573593133701));
#19254=CARTESIAN_POINT('Origin',(-200.579725765336,169.864132597105,276.573593133701));
#19255=CARTESIAN_POINT('',(-201.000801525488,178.301963356951,234.573593133701));
#19256=CARTESIAN_POINT('',(-203.720171215434,232.794725440707,234.573593133701));
#19257=CARTESIAN_POINT('',(-198.088104690518,119.935167464172,234.573593133701));
#19258=CARTESIAN_POINT('',(-201.000801525488,178.301963356951,276.573593133701));
#19259=CARTESIAN_POINT('Origin',(-204.966203632451,257.763654196578,237.573593133701));
#19260=CARTESIAN_POINT('Origin',(-204.966203632451,257.763654196578,268.573593133701));
#19261=CARTESIAN_POINT('',(-201.000801525488,178.301963356951,271.573593133701));
#19262=CARTESIAN_POINT('',(-201.000801525488,178.301963356951,276.573593133701));
#19263=CARTESIAN_POINT('',(-203.720171215434,232.794725440707,271.573593133701));
#19264=CARTESIAN_POINT('',(-203.720171215434,232.794725440707,271.573593133701));
#19265=CARTESIAN_POINT('',(-203.720171215434,232.794725440707,234.573593133701));
#19266=CARTESIAN_POINT('',(-203.969377698837,237.788511191881,234.573593133701));
#19267=CARTESIAN_POINT('',(-203.969377698837,237.788511191881,234.573593133701));
#19268=CARTESIAN_POINT('',(-203.969377698837,237.788511191881,271.573593133701));
#19269=CARTESIAN_POINT('',(-203.969377698837,237.788511191881,271.573593133701));
#19270=CARTESIAN_POINT('',(-204.966203632451,257.763654196578,271.573593133701));
#19271=CARTESIAN_POINT('',(-205.115727522493,260.759925647282,237.573593133701));
#19272=CARTESIAN_POINT('Origin',(-204.966203632451,257.763654196578,237.573593133701));
#19273=CARTESIAN_POINT('Origin',(-262.39258353924,254.897887240558,268.573593133701));
#19274=CARTESIAN_POINT('Origin',(-276.127908375746,229.181339034477,234.573593133701));
#19275=CARTESIAN_POINT('',(-276.127908375746,229.181339034477,234.573593133701));
#19276=CARTESIAN_POINT('',(-276.127908375746,229.181339034477,271.573593133701));
#19277=CARTESIAN_POINT('Origin',(-270.49584185083,116.321781057942,234.573593133701));
#19278=CARTESIAN_POINT('Origin',(-220.975944530184,177.305137423337,234.573593133701));
#19279=CARTESIAN_POINT('Origin',(-280.877471090321,173.835684387434,234.573593133701));
#19280=CARTESIAN_POINT('Origin',(-276.127908375746,229.181339034477,271.573593133701));
#19281=CARTESIAN_POINT('Origin',(-220.975944530184,177.305137423337,271.573593133701));
#19282=CARTESIAN_POINT('Origin',(-280.877471090321,173.835684387434,271.573593133701));
#19283=CARTESIAN_POINT('Origin',(-276.377114859149,234.175124785651,271.573593133701));
#19284=CARTESIAN_POINT('',(-276.377114859149,234.175124785651,271.573593133701));
#19285=CARTESIAN_POINT('',(-276.377114859149,234.175124785651,234.573593133701));
#19286=CARTESIAN_POINT('Origin',(-277.373940792763,254.150267790348,271.573593133701));
#19287=CARTESIAN_POINT('Origin',(-277.523464682805,257.146539241052,237.573593133701));
#19288=CARTESIAN_POINT('Origin',(-276.377114859149,234.175124785651,234.573593133701));
#19289=CARTESIAN_POINT('Origin',(-235.078442029538,259.264686746862,253.073593133701));
#19290=CARTESIAN_POINT('Origin',(-234.829235546134,254.270900995688,253.073593133701));
#19291=CARTESIAN_POINT('Origin',(-280.877471090321,173.835684387434,276.573593133701));
#19292=CARTESIAN_POINT('Origin',(-280.877471090321,173.835684387434,276.573593133701));
#19293=CARTESIAN_POINT('Origin',(-220.975944530184,177.305137423337,276.573593133701));
#19294=CARTESIAN_POINT('Origin',(-220.975944530184,177.305137423337,276.573593133701));
#27757=UNCERTAINTY_MEASURE_WITH_UNIT(LENGTH_MEASURE(0.01),#27808,
'DISTANCE_ACCURACY_VALUE',
'Maximum model space distance between geometric entities at asserted c
onnectivities');
#27778=UNCERTAINTY_MEASURE_WITH_UNIT(LENGTH_MEASURE(0.01),#27808,
'DISTANCE_ACCURACY_VALUE',
'Maximum model space distance between geometric entities at asserted c
onnectivities');
#27786=(
GEOMETRIC_REPRESENTATION_CONTEXT(3)
GLOBAL_UNCERTAINTY_ASSIGNED_CONTEXT((#27757))
GLOBAL_UNIT_ASSIGNED_CONTEXT((#27808,#27810,#27811))
REPRESENTATION_CONTEXT('','3D')
);
#27807=(
GEOMETRIC_REPRESENTATION_CONTEXT(3)
GLOBAL_UNCERTAINTY_ASSIGNED_CONTEXT((#27778))
GLOBAL_UNIT_ASSIGNED_CONTEXT((#27808,#27810,#27811))
REPRESENTATION_CONTEXT('','3D')
);
#27808=(
LENGTH_UNIT()
NAMED_UNIT(*)
SI_UNIT(.MILLI.,.METRE.)
);
#27810=(
NAMED_UNIT(*)
PLANE_ANGLE_UNIT()
SI_UNIT($,.RADIAN.)
);
#27811=(
NAMED_UNIT(*)
SI_UNIT($,.STERADIAN.)
SOLID_ANGLE_UNIT()
);
#27819=SHAPE_DEFINITION_REPRESENTATION(#27849,#27906);
#27849=PRODUCT_DEFINITION_SHAPE('',$,#27935);
#27906=SHAPE_REPRESENTATION('',(#12859),#27786);
#27927=PRODUCT_DEFINITION_CONTEXT('part definition',#28013,'design');
#27935=PRODUCT_DEFINITION('Saddle Holder','Saddle Holder',#27963,#27927);
#27963=PRODUCT_DEFINITION_FORMATION('',$,#28022);
#28013=APPLICATION_CONTEXT('Managed model based 3d engineering');
#28014=PRODUCT_CONTEXT('part definition',#28013,'mechanical');
#28022=PRODUCT('Saddle Holder','Saddle Holder',$,(#28014));
#28085=COLOUR_RGB('Off White',0.89,0.88,0.83);
#28086=FILL_AREA_STYLE_COLOUR('',#28085);
#28087=FILL_AREA_STYLE('',(#28086));
#28088=SURFACE_STYLE_FILL_AREA(#28087);
#28089=SURFACE_SIDE_STYLE('',(#28088));
#28090=SURFACE_STYLE_USAGE(.BOTH.,#28089);
#28091=PRESENTATION_STYLE_ASSIGNMENT((#28090));
ENDSEC;
END-ISO-10303-21;
